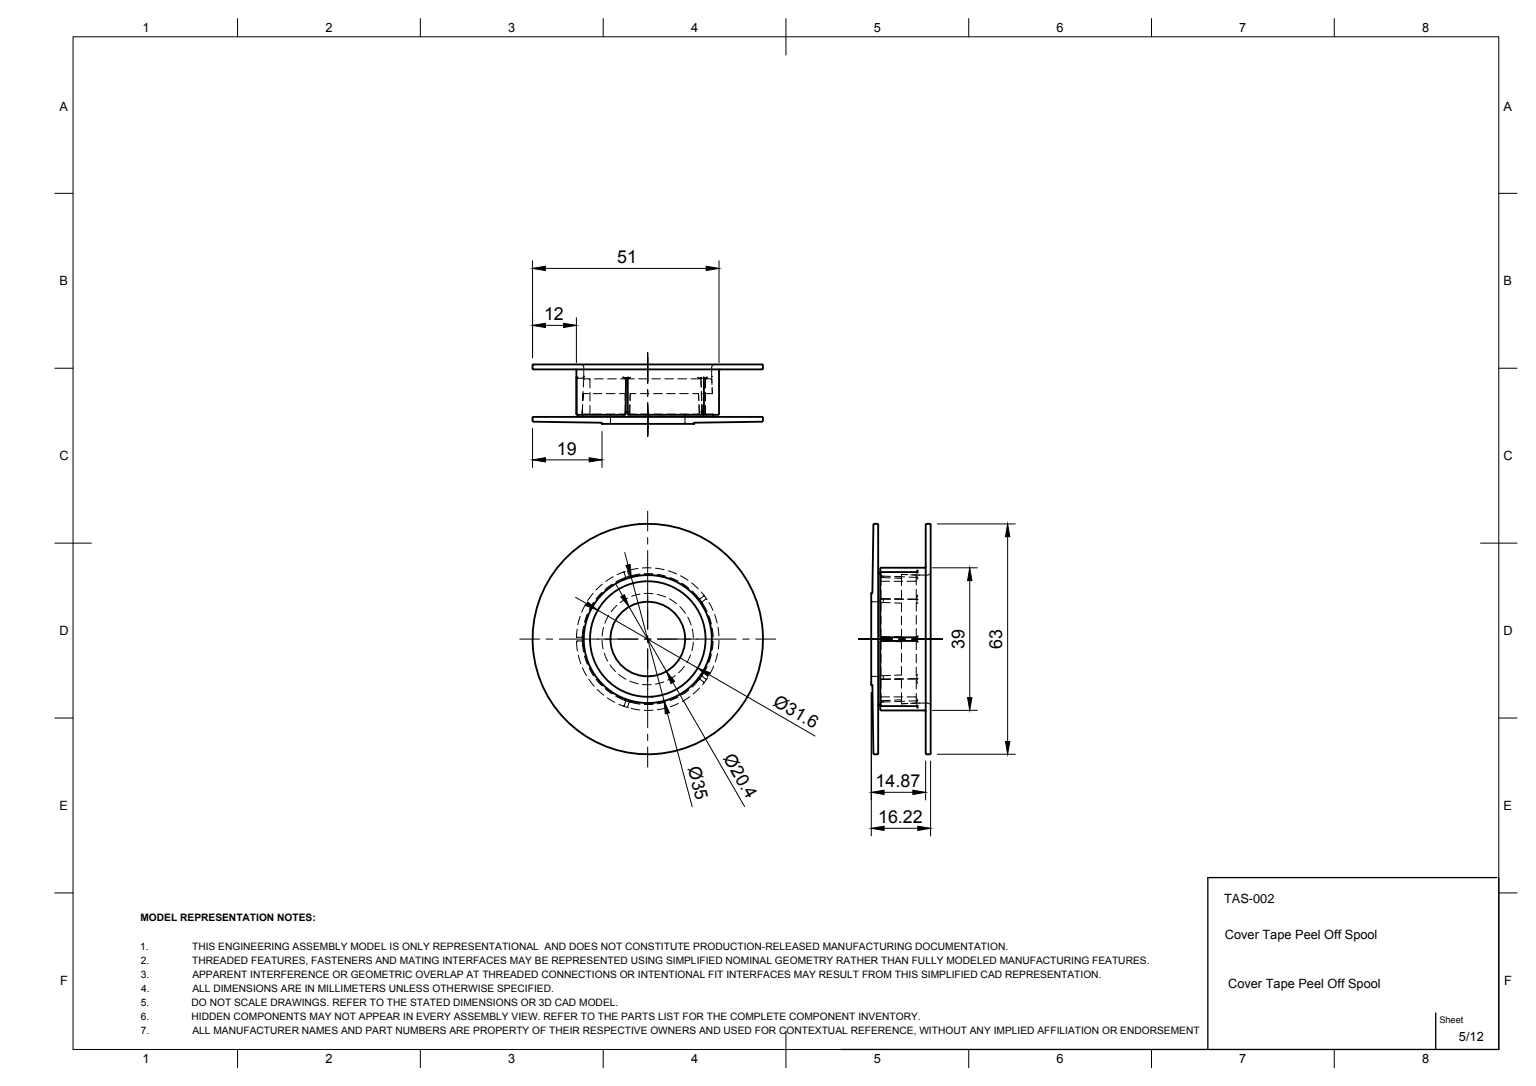
ISO-10303-21;
HEADER;
/* Generated by software containing ST-Developer
 * from STEP Tools, Inc. (www.steptools.com) 
 */

FILE_DESCRIPTION(
/* description */ ('STEP AP214'),
/* implementation_level */ '2;1');

FILE_NAME(
/* name */ 'Cover Tape Peel Off Spool.step',
/* time_stamp */ '2026-11-04T19:38:14-08:00',
/* author */ (''),
/* organization */ (''),
/* preprocessor_version */ 'ST-DEVELOPER v20.2',
/* originating_system */ 'Autodesk Translation Framework v15.17.0.0',
/* authorisation */ '');

FILE_SCHEMA (('AUTOMOTIVE_DESIGN { 1 0 10303 214 3 1 1 }'));
ENDSEC;

DATA;
#10=MECHANICAL_DESIGN_GEOMETRIC_PRESENTATION_REPRESENTATION('',(#472),#36668);
#168=CONICAL_SURFACE('',#18363,17.5,0.0444152152469099);
#169=CONICAL_SURFACE('',#18378,31.5,1.55500816505907);
#170=CONICAL_SURFACE('',#18555,17.5,0.038076825589802);
#193=TOROIDAL_SURFACE('',#18311,15.5,0.3);
#194=TOROIDAL_SURFACE('',#18315,31.2,0.3);
#195=TOROIDAL_SURFACE('',#18320,12.8,0.3);
#196=TOROIDAL_SURFACE('',#18325,10.5,0.3);
#197=TOROIDAL_SURFACE('',#18329,10.5,0.3);
#198=TOROIDAL_SURFACE('',#18334,31.2,0.3);
#199=TOROIDAL_SURFACE('',#18338,18.2,0.3);
#200=TOROIDAL_SURFACE('',#18342,17.2130371832119,0.3);
#201=TOROIDAL_SURFACE('',#18346,16.1,0.3);
#202=TOROIDAL_SURFACE('',#18380,31.25,0.25);
#203=TOROIDAL_SURFACE('',#18385,19.75,0.25);
#204=TOROIDAL_SURFACE('',#18389,17.75,0.25);
#205=TOROIDAL_SURFACE('',#18399,18.1406575306034,0.25);
#206=TOROIDAL_SURFACE('',#18405,19.25,0.25);
#207=TOROIDAL_SURFACE('',#18411,17.759705149651,0.25);
#208=TOROIDAL_SURFACE('',#18414,19.25,0.25);
#209=TOROIDAL_SURFACE('',#18425,17.759705149651,0.25);
#210=TOROIDAL_SURFACE('',#18431,19.25,0.25);
#211=TOROIDAL_SURFACE('',#18435,18.1406575306034,0.25);
#212=TOROIDAL_SURFACE('',#18439,19.25,0.25);
#213=TOROIDAL_SURFACE('',#18452,18.1406575306034,0.25);
#214=TOROIDAL_SURFACE('',#18458,19.25,0.25);
#215=TOROIDAL_SURFACE('',#18462,17.759705149651,0.25);
#216=TOROIDAL_SURFACE('',#18465,19.25,0.25);
#217=TOROIDAL_SURFACE('',#18479,17.759705149651,0.25);
#218=TOROIDAL_SURFACE('',#18485,19.25,0.25);
#219=TOROIDAL_SURFACE('',#18490,18.1406575306034,0.25);
#220=TOROIDAL_SURFACE('',#18493,19.25,0.25);
#221=TOROIDAL_SURFACE('',#18506,18.1406575306034,0.25);
#222=TOROIDAL_SURFACE('',#18513,19.25,0.25);
#223=TOROIDAL_SURFACE('',#18520,17.759705149651,0.25);
#224=TOROIDAL_SURFACE('',#18523,19.25,0.25);
#225=TOROIDAL_SURFACE('',#18530,31.25,0.25);
#226=TOROIDAL_SURFACE('',#18551,18.2999999294072,0.8);
#236=B_SPLINE_CURVE_WITH_KNOTS('',3,(#25581,#25582,#25583,#25584,#25585,
#25586,#25587,#25588,#25589,#25590,#25591,#25592),.UNSPECIFIED.,.F.,.F.,
(4,2,2,2,2,4),(-0.0307505677232343,-0.0290851658458097,-0.0274197639683852,
-0.0256899175968281,-0.0239600712252709,-0.0214016072500974),
 .UNSPECIFIED.);
#237=B_SPLINE_CURVE_WITH_KNOTS('',3,(#25608,#25609,#25610,#25611,#25612,
#25613,#25614,#25615,#25616,#25617,#25618,#25619),.UNSPECIFIED.,.F.,.F.,
(4,2,2,2,2,4),(-0.0400996909613273,-0.0375410642212333,-0.035811217849675,
-0.0340813714781167,-0.0324159696006892,-0.0307505677232617),
 .UNSPECIFIED.);
#238=B_SPLINE_CURVE_WITH_KNOTS('',3,(#25634,#25635,#25636,#25637,#25638,
#25639,#25640,#25641,#25642,#25643,#25644,#25645),.UNSPECIFIED.,.F.,.F.,
(4,2,2,2,2,4),(0.0307505677231893,0.0324159696006138,0.0340813714780383,
0.0358112178495909,0.0375410642211435,0.040099528194227),.UNSPECIFIED.);
#239=B_SPLINE_CURVE_WITH_KNOTS('',3,(#25652,#25653,#25654,#25655,#25656,
#25657,#25658,#25659,#25660,#25661,#25662,#25663),.UNSPECIFIED.,.F.,.F.,
(4,2,2,2,2,4),(0.0214015561623852,0.0239600712252435,0.0256899175967988,
0.0274197639683542,0.0290851658457769,0.0307505677231996),.UNSPECIFIED.);
#240=B_SPLINE_CURVE_WITH_KNOTS('',3,(#25749,#25750,#25751,#25752,#25753,
#25754,#25755,#25756,#25757,#25758,#25759,#25760),.UNSPECIFIED.,.F.,.F.,
(4,2,2,2,2,4),(0.0214014871422872,0.0239600712252674,0.0256899175968258,
0.0274197639683841,0.0290851658458094,0.0307505677232346),.UNSPECIFIED.);
#241=B_SPLINE_CURVE_WITH_KNOTS('',3,(#25762,#25763,#25764,#25765,#25766,
#25767),.UNSPECIFIED.,.F.,.F.,(4,2,4),(0.516167584835576,0.556355629697994,
0.571945746029783),.UNSPECIFIED.);
#242=B_SPLINE_CURVE_WITH_KNOTS('',3,(#25770,#25771,#25772,#25773,#25774,
#25775),.UNSPECIFIED.,.F.,.F.,(4,2,4),(-0.572283818814118,-0.556572033620994,
-0.516504886359884),.UNSPECIFIED.);
#243=B_SPLINE_CURVE_WITH_KNOTS('',3,(#25778,#25779,#25780,#25781,#25782,
#25783),.UNSPECIFIED.,.F.,.F.,(4,2,4),(0.516062927236787,0.556286483365537,
0.571840801367595),.UNSPECIFIED.);
#244=B_SPLINE_CURVE_WITH_KNOTS('',3,(#25787,#25788,#25789,#25790,#25791,
#25792),.UNSPECIFIED.,.F.,.F.,(4,2,4),(-0.572388774164482,-0.556641170070289,
-0.516609564275015),.UNSPECIFIED.);
#245=B_SPLINE_CURVE_WITH_KNOTS('',3,(#25794,#25795,#25796,#25797,#25798,
#25799,#25800,#25801,#25802,#25803,#25804,#25805),.UNSPECIFIED.,.F.,.F.,
(4,2,2,2,2,4),(0.0307505677232594,0.0324159696006859,0.0340813714781124,
0.0358112178496696,0.0375410642212269,0.0400994853939697),.UNSPECIFIED.);
#246=B_SPLINE_CURVE_WITH_KNOTS('',3,(#25809,#25810,#25811,#25812,#25813,
#25814,#25815,#25816,#25817,#25818,#25819,#25820),.UNSPECIFIED.,.F.,.F.,
(4,2,2,2,2,4),(0.0214014871425106,0.0239600712253013,0.0256899175968606,
0.0274197639684198,0.0290851658458467,0.0307505677232736),.UNSPECIFIED.);
#247=B_SPLINE_CURVE_WITH_KNOTS('',3,(#25822,#25823,#25824,#25825,#25826,
#25827),.UNSPECIFIED.,.F.,.F.,(4,2,4),(0.516167584819259,0.556355629663768,
0.571945746013171),.UNSPECIFIED.);
#248=B_SPLINE_CURVE_WITH_KNOTS('',3,(#25830,#25831,#25832,#25833,#25834,
#25835),.UNSPECIFIED.,.F.,.F.,(4,2,4),(-0.572283818796558,-0.556572033600684,
-0.516504886344356),.UNSPECIFIED.);
#249=B_SPLINE_CURVE_WITH_KNOTS('',3,(#25839,#25840,#25841,#25842,#25843,
#25844,#25845,#25846,#25847,#25848,#25849,#25850),.UNSPECIFIED.,.F.,.F.,
(4,2,2,2,2,4),(0.0214015561620376,0.0239600712252775,0.0256899175968367,
0.0274197639683959,0.0290851658458218,0.0307505677232477),.UNSPECIFIED.);
#250=B_SPLINE_CURVE_WITH_KNOTS('',3,(#25852,#25853,#25854,#25855,#25856,
#25857),.UNSPECIFIED.,.F.,.F.,(4,2,4),(0.516336929306378,0.556467476401172,
0.572115549692269),.UNSPECIFIED.);
#251=B_SPLINE_CURVE_WITH_KNOTS('',3,(#25861,#25862,#25863,#25864,#25865,
#25866),.UNSPECIFIED.,.F.,.F.,(4,2,4),(-0.572113997134204,-0.556460133617456,
-0.516335518817303),.UNSPECIFIED.);
#252=B_SPLINE_CURVE_WITH_KNOTS('',3,(#25868,#25869,#25870,#25871,#25872,
#25873,#25874,#25875,#25876,#25877,#25878,#25879),.UNSPECIFIED.,.F.,.F.,
(4,2,2,2,2,4),(0.0307505677232669,0.0324159696006922,0.0340813714781176,
0.0358112178496757,0.0375410642212338,0.0400995974505249),.UNSPECIFIED.);
#253=B_SPLINE_CURVE_WITH_KNOTS('',3,(#25882,#25883,#25884,#25885,#25886,
#25887),.UNSPECIFIED.,.F.,.F.,(4,2,4),(0.516336929316142,0.556467476363535,
0.572115549701707),.UNSPECIFIED.);
#254=B_SPLINE_CURVE_WITH_KNOTS('',3,(#25891,#25892,#25893,#25894,#25895,
#25896),.UNSPECIFIED.,.F.,.F.,(4,2,4),(-0.572087843455165,-0.556460133653863,
-0.516335518814487),.UNSPECIFIED.);
#255=B_SPLINE_CURVE_WITH_KNOTS('',3,(#25898,#25899,#25900,#25901,#25902,
#25903,#25904,#25905,#25906,#25907,#25908,#25909),.UNSPECIFIED.,.F.,.F.,
(4,2,2,2,2,4),(0.0307505677231587,0.0324159696005802,0.0340813714780017,
0.0358112178495531,0.0375410642211044,0.0401277329731923),.UNSPECIFIED.);
#256=B_SPLINE_CURVE_WITH_KNOTS('',3,(#25915,#25916,#25917,#25918,#25919,
#25920,#25921,#25922,#25923,#25924,#25925,#25926,#25927,#25928,#25929,#25930,
#25931,#25932,#25933,#25934,#25935,#25936),.UNSPECIFIED.,.F.,.F.,(4,2,2,
2,2,2,2,2,2,2,4),(2.02457825278125E-10,0.00248408483075073,0.00372612724612612,
0.00434714845381382,0.00465765905765771,0.00481291435957969,0.00489054201054069,
0.00492935583602118,0.00494876274876143,0.00495846620513155,0.00496816966150168),
 .UNSPECIFIED.);
#257=B_SPLINE_CURVE_WITH_KNOTS('',3,(#25938,#25939,#25940,#25941,#25942,
#25943,#25944,#25945,#25946,#25947,#25948,#25949,#25950,#25951,#25952,#25953,
#25954,#25955,#25956,#25957,#25958,#25959),.UNSPECIFIED.,.F.,.F.,(4,2,2,
2,2,2,2,2,2,2,4),(3.5048712953905E-5,4.4761383731225E-5,5.4474054508545E-5,
7.38993960631036E-5,0.00011275007917231,0.000190451445390804,0.000345854177827798,
0.000656659642701783,0.00127827057244967,0.00252149243194545,0.00500793615093709),
 .UNSPECIFIED.);
#258=B_SPLINE_CURVE_WITH_KNOTS('',3,(#25962,#25963,#25964,#25965,#25966,
#25967,#25968,#25969,#25970,#25971,#25972,#25973,#25974,#25975,#25976,#25977,
#25978,#25979,#25980,#25981,#25982,#25983),.UNSPECIFIED.,.F.,.F.,(4,2,2,
2,2,2,2,2,2,2,4),(2.04137276529534E-10,0.00248408522863344,0.00372612784295016,
0.00434714915010856,0.00465765980368776,0.00481291513047741,0.00489054279387223,
0.00492935662556968,0.00494876354141844,0.00495846699934282,0.0049681704572672),
 .UNSPECIFIED.);
#259=B_SPLINE_CURVE_WITH_KNOTS('',3,(#25985,#25986,#25987,#25988,#25989,
#25990,#25991,#25992,#25993,#25994,#25995,#25996,#25997,#25998,#25999,#26000,
#26001,#26002,#26003,#26004,#26005,#26006),.UNSPECIFIED.,.F.,.F.,(4,2,2,
2,2,2,2,2,2,2,4),(3.50520341719619E-5,4.47649965919165E-5,5.44779590118712E-5,
7.3903883851858E-5,0.000112755733531832,0.0001904594328917,0.000345866831611521,
0.000656681629051249,0.00127831122393071,0.00252157041368962,0.00500808879320745),
 .UNSPECIFIED.);
#260=B_SPLINE_CURVE_WITH_KNOTS('',3,(#26014,#26015,#26016,#26017,#26018,
#26019,#26020,#26021,#26022,#26023,#26024,#26025,#26026,#26027,#26028,#26029,
#26030,#26031,#26032,#26033,#26034,#26035),.UNSPECIFIED.,.F.,.F.,(4,2,2,
2,2,2,2,2,2,2,4),(2.06866606511861E-10,0.00248408587267595,0.00372612880901388,
0.00434715027718289,0.00465766101126744,0.00481291637830975,0.00489054406183091,
0.00492935790359148,0.00494876482447177,0.00495846828491192,0.00496817174535206),
 .UNSPECIFIED.);
#261=B_SPLINE_CURVE_WITH_KNOTS('',3,(#26037,#26038,#26039,#26040,#26041,
#26042,#26043,#26044,#26045,#26046,#26047,#26048,#26049,#26050,#26051,#26052,
#26053,#26054,#26055,#26056,#26057,#26058),.UNSPECIFIED.,.F.,.F.,(4,2,2,
2,2,2,2,2,2,2,4),(3.50574081053878E-5,4.47708507809905E-5,5.44842934565933E-5,
7.39111788077861E-5,0.000112764949510167,0.000190472490915007,0.000345887573724691,
0.000656717739344059,0.00127837807058271,0.00252169873306001,0.00500834005801461),
 .UNSPECIFIED.);
#262=B_SPLINE_CURVE_WITH_KNOTS('',3,(#26061,#26062,#26063,#26064,#26065,
#26066,#26067,#26068,#26069,#26070,#26071,#26072,#26073,#26074,#26075,#26076,
#26077,#26078,#26079,#26080,#26081,#26082),.UNSPECIFIED.,.F.,.F.,(4,2,2,
2,2,2,2,2,2,2,4),(2.06867445612259E-10,0.00248408587267104,0.00372612880900657,
0.00434715027717433,0.00465766101125817,0.00481291637830013,0.00489054406182111,
0.0049293579035816,0.00494876482446188,0.00495846828490199,0.00496817174534209),
 .UNSPECIFIED.);
#263=B_SPLINE_CURVE_WITH_KNOTS('',3,(#26084,#26085,#26086,#26087,#26088,
#26089,#26090,#26091,#26092,#26093,#26094,#26095,#26096,#26097,#26098,#26099,
#26100,#26101,#26102,#26103,#26104,#26105),.UNSPECIFIED.,.F.,.F.,(4,2,2,
2,2,2,2,2,2,2,4),(3.50574081266199E-5,4.47708505998206E-5,5.44842930730214E-5,
7.39111780194308E-5,0.000112764947912246,0.000190472487697963,0.000345887567269397,
0.000656717726412263,0.001278378044698,0.00252169868126955,0.00500833995441257),
 .UNSPECIFIED.);
#264=B_SPLINE_CURVE_WITH_KNOTS('',3,(#26108,#26109,#26110,#26111,#26112,
#26113,#26114,#26115,#26116,#26117,#26118,#26119,#26120,#26121,#26122,#26123,
#26124,#26125,#26126,#26127,#26128,#26129),.UNSPECIFIED.,.F.,.F.,(4,2,2,
2,2,2,2,2,2,2,4),(2.04137059199594E-10,0.00248408522863389,0.00372612784295087,
0.00434714915010935,0.00465765980368859,0.00481291513047817,0.00489054279387297,
0.00492935662557032,0.00494876354141895,0.00495846699934332,0.00496817045726768),
 .UNSPECIFIED.);
#265=B_SPLINE_CURVE_WITH_KNOTS('',3,(#26130,#26131,#26132,#26133,#26134,
#26135,#26136,#26137,#26138,#26139,#26140,#26141,#26142,#26143,#26144,#26145,
#26146,#26147,#26148,#26149,#26150,#26151),.UNSPECIFIED.,.F.,.F.,(4,2,2,
2,2,2,2,2,2,2,4),(3.50520341720812E-5,4.47649965026772E-5,5.44779588332732E-5,
7.39038834943838E-5,0.000112755732816681,0.00019045943146128,0.000345866828750562,
0.00065668162332904,0.00127831121248599,0.00252157039079989,0.00500808874742778),
 .UNSPECIFIED.);
#266=B_SPLINE_CURVE_WITH_KNOTS('',3,(#26205,#26206,#26207,#26208,#26209,
#26210,#26211,#26212,#26213,#26214,#26215,#26216,#26217,#26218),
 .UNSPECIFIED.,.F.,.F.,(4,2,2,2,2,2,4),(-0.000304965314045538,0.,0.000936499595052828,
0.00576011793928687,0.00947606916598535,0.0122802204486003,0.0139854910646116),
 .UNSPECIFIED.);
#267=B_SPLINE_CURVE_WITH_KNOTS('',3,(#26225,#26226,#26227,#26228,#26229,
#26230,#26231,#26232,#26233,#26234,#26235,#26236,#26237,#26238,#26239,#26240),
 .UNSPECIFIED.,.F.,.F.,(4,2,2,2,2,2,2,4),(0.0536858997421767,0.0538805473387552,
0.0625727109542441,0.0725640535967514,0.0859159770081403,0.0987536985065928,
0.112218387900172,0.112607088674662),.UNSPECIFIED.);
#268=B_SPLINE_CURVE_WITH_KNOTS('',3,(#26255,#26256,#26257,#26258,#26259,
#26260,#26261,#26262,#26263,#26264,#26265,#26266,#26267,#26268,#26269,#26270),
 .UNSPECIFIED.,.F.,.F.,(4,2,2,2,2,2,2,4),(-0.0122740412193648,-0.0121759293582432,
-0.0120897396500415,-0.0111319415843575,-0.00947389246986148,-0.00820108783558479,
-0.0071868786468098,-0.00688693855294442),.UNSPECIFIED.);
#269=B_SPLINE_CURVE_WITH_KNOTS('',3,(#26276,#26277,#26278,#26279,#26280,
#26281,#26282,#26283,#26284,#26285,#26286,#26287,#26288,#26289,#26290,#26291),
 .UNSPECIFIED.,.F.,.F.,(4,2,2,2,2,2,2,4),(-0.0477691295327812,-0.0476102750821729,
-0.0405164866112679,-0.0323624211355981,-0.0214657417184032,-0.0109887092110674,
0.,0.000317223788085325),.UNSPECIFIED.);
#270=B_SPLINE_CURVE_WITH_KNOTS('',3,(#26303,#26304,#26305,#26306,#26307,
#26308,#26309,#26310,#26311,#26312,#26313,#26314,#26315,#26316,#26317,#26318),
 .UNSPECIFIED.,.F.,.F.,(4,2,2,2,2,2,2,4),(0.00685142344086609,0.00716754606670829,
0.00817883021840179,0.00945159950065682,0.0111102560598908,0.0126000677878647,
0.0134555802450022,0.0143116650403246),.UNSPECIFIED.);
#271=B_SPLINE_CURVE_WITH_KNOTS('',3,(#26340,#26341,#26342,#26343,#26344,
#26345,#26346,#26347,#26348,#26349,#26350,#26351,#26352,#26353,#26354,#26355),
 .UNSPECIFIED.,.F.,.F.,(4,2,2,2,2,2,2,4),(-0.000317223787690337,3.02215934569472E-15,
0.0109887092111399,0.0214657417185508,0.0323624211357588,0.0405164866114483,
0.0476102750823548,0.047769129532989),.UNSPECIFIED.);
#272=B_SPLINE_CURVE_WITH_KNOTS('',3,(#26359,#26360,#26361,#26362,#26363,
#26364,#26365,#26366,#26367,#26368,#26369,#26370,#26371,#26372),
 .UNSPECIFIED.,.F.,.F.,(4,2,2,2,2,2,4),(-0.0138875980614929,-0.0121989286884961,
-0.00941634599982081,-0.00572975137256096,-0.00094390537822651,0.,0.000305060128611046),
 .UNSPECIFIED.);
#273=B_SPLINE_CURVE_WITH_KNOTS('',3,(#26384,#26385,#26386,#26387,#26388,
#26389,#26390,#26391,#26392,#26393,#26394,#26395,#26396,#26397,#26398,#26399),
 .UNSPECIFIED.,.F.,.F.,(4,2,2,2,2,2,2,4),(-0.112607088625168,-0.112218387851368,
-0.0987536984648267,-0.0859159769729998,-0.0725640535676872,-0.0625727109298437,
-0.0538805473185267,-0.053685899721448),.UNSPECIFIED.);
#274=B_SPLINE_CURVE_WITH_KNOTS('',3,(#26440,#26441,#26442,#26443,#26444,
#26445,#26446,#26447,#26448,#26449,#26450,#26451,#26452,#26453),
 .UNSPECIFIED.,.F.,.F.,(4,2,2,2,2,2,4),(-0.000304965268692175,0.,0.000936496117482782,
0.00576013224595397,0.00947609729856078,0.0122802587445126,0.0139855371807907),
 .UNSPECIFIED.);
#275=B_SPLINE_CURVE_WITH_KNOTS('',3,(#26463,#26464,#26465,#26466,#26467,
#26468,#26469,#26470,#26471,#26472,#26473,#26474,#26475,#26476,#26477,#26478),
 .UNSPECIFIED.,.F.,.F.,(4,2,2,2,2,2,2,4),(0.0536858997392164,0.0538805473358447,
0.0625727109506776,0.072564053592395,0.0859159770028611,0.0987536985002761,
0.112218387892815,0.112607088666955),.UNSPECIFIED.);
#276=B_SPLINE_CURVE_WITH_KNOTS('',3,(#26492,#26493,#26494,#26495,#26496,
#26497,#26498,#26499,#26500,#26501,#26502,#26503,#26504,#26505,#26506,#26507),
 .UNSPECIFIED.,.F.,.F.,(4,2,2,2,2,2,2,4),(-0.0122740769336355,-0.0121759644410632,
-0.0120897737524462,-0.0111319575392944,-0.00947390765146132,-0.00820110219546828,
-0.00718689112173828,-0.00688695772759274),.UNSPECIFIED.);
#277=B_SPLINE_CURVE_WITH_KNOTS('',3,(#26513,#26514,#26515,#26516,#26517,
#26518,#26519,#26520,#26521,#26522,#26523,#26524,#26525,#26526,#26527,#26528),
 .UNSPECIFIED.,.F.,.F.,(4,2,2,2,2,2,2,4),(-0.0477691295328705,-0.0476102750818484,
-0.0405164866108641,-0.0323624211350328,-0.0214657417175428,-0.0109887092105592,
0.,0.00031722378862325),.UNSPECIFIED.);
#278=B_SPLINE_CURVE_WITH_KNOTS('',3,(#26544,#26545,#26546,#26547,#26548,
#26549,#26550,#26551,#26552,#26553,#26554,#26555,#26556,#26557,#26558,#26559),
 .UNSPECIFIED.,.F.,.F.,(4,2,2,2,2,2,2,4),(0.00683098498387795,0.00715685727468737,
0.0081665770863791,0.0094395668715797,0.0110988523787266,0.0125271081563038,
0.0131709865966103,0.0138210554549785),.UNSPECIFIED.);
#279=B_SPLINE_CURVE_WITH_KNOTS('',3,(#26580,#26581,#26582,#26583,#26584,
#26585,#26586,#26587,#26588,#26589,#26590,#26591,#26592,#26593,#26594,#26595),
 .UNSPECIFIED.,.F.,.F.,(4,2,2,2,2,2,2,4),(-0.000317223788318669,0.,0.0109887092111283,
0.0214657417185403,0.0323624211358337,0.0405164866115566,0.0476102750824874,
0.0477691295331555),.UNSPECIFIED.);
#280=B_SPLINE_CURVE_WITH_KNOTS('',3,(#26599,#26600,#26601,#26602,#26603,
#26604,#26605,#26606,#26607,#26608,#26609,#26610,#26611,#26612),
 .UNSPECIFIED.,.F.,.F.,(4,2,2,2,2,2,4),(-0.013826978099047,-0.0121485991715528,
-0.00937937937785604,-0.00571097373361621,-0.000948519651099016,0.,0.00030511843446065),
 .UNSPECIFIED.);
#281=B_SPLINE_CURVE_WITH_KNOTS('',3,(#26624,#26625,#26626,#26627,#26628,
#26629,#26630,#26631,#26632,#26633,#26634,#26635,#26636,#26637,#26638,#26639),
 .UNSPECIFIED.,.F.,.F.,(4,2,2,2,2,2,2,4),(-0.112607088663875,-0.112218387889847,
-0.0987536984976824,-0.0859159770006442,-0.0725640535905707,-0.0625727109491047,
-0.0538805473344791,-0.0536858997378307),.UNSPECIFIED.);
#282=B_SPLINE_CURVE_WITH_KNOTS('',3,(#26682,#26683,#26684,#26685,#26686,
#26687,#26688,#26689,#26690,#26691,#26692,#26693,#26694,#26695),
 .UNSPECIFIED.,.F.,.F.,(4,2,2,2,2,2,4),(-0.00030506004969664,0.,0.000943899264666623,
0.00572977625979271,0.0094163950019481,0.012198995415075,0.0138876784363644),
 .UNSPECIFIED.);
#283=B_SPLINE_CURVE_WITH_KNOTS('',3,(#26705,#26706,#26707,#26708,#26709,
#26710,#26711,#26712,#26713,#26714,#26715,#26716,#26717,#26718,#26719,#26720),
 .UNSPECIFIED.,.F.,.F.,(4,2,2,2,2,2,2,4),(0.0536858997405358,0.053880547337153,
0.0625727109524208,0.072564053594619,0.0859159770056253,0.0987536985036731,
0.112218387896803,0.112607088671311),.UNSPECIFIED.);
#284=B_SPLINE_CURVE_WITH_KNOTS('',3,(#26737,#26738,#26739,#26740,#26741,
#26742,#26743,#26744,#26745,#26746,#26747,#26748,#26749,#26750,#26751,#26752),
 .UNSPECIFIED.,.F.,.F.,(4,2,2,2,2,2,2,4),(-0.0143120844458313,-0.0134558136848229,
-0.0126001113738633,-0.0111102618619966,-0.00945160573383406,-0.00817883662994094,
-0.00716755165087691,-0.00685143448301955),.UNSPECIFIED.);
#285=B_SPLINE_CURVE_WITH_KNOTS('',3,(#26758,#26759,#26760,#26761,#26762,
#26763,#26764,#26765,#26766,#26767,#26768,#26769,#26770,#26771,#26772,#26773),
 .UNSPECIFIED.,.F.,.F.,(4,2,2,2,2,2,2,4),(-0.0477691295329166,-0.0476102750829768,
-0.0405164866121143,-0.0323624211366189,-0.0214657417197341,-0.0109887092118291,
0.,0.000317223787610884),.UNSPECIFIED.);
#387=SPHERICAL_SURFACE('',#18271,0.25);
#388=SPHERICAL_SURFACE('',#18275,0.25);
#389=SPHERICAL_SURFACE('',#18279,0.25);
#390=SPHERICAL_SURFACE('',#18283,0.25);
#391=SPHERICAL_SURFACE('',#18287,0.25);
#392=SPHERICAL_SURFACE('',#18291,0.25);
#393=SPHERICAL_SURFACE('',#18295,0.25);
#394=SPHERICAL_SURFACE('',#18299,0.25);
#395=SPHERICAL_SURFACE('',#18303,0.25);
#396=SPHERICAL_SURFACE('',#18307,0.25);
#397=SPHERICAL_SURFACE('',#18396,0.25);
#398=SPHERICAL_SURFACE('',#18408,0.25);
#399=SPHERICAL_SURFACE('',#18428,0.25);
#400=SPHERICAL_SURFACE('',#18445,0.25);
#401=SPHERICAL_SURFACE('',#18448,0.25);
#402=SPHERICAL_SURFACE('',#18468,0.25);
#403=SPHERICAL_SURFACE('',#18482,0.25);
#404=SPHERICAL_SURFACE('',#18499,0.25);
#405=SPHERICAL_SURFACE('',#18502,0.25);
#406=SPHERICAL_SURFACE('',#18517,0.25);
#452=SHAPE_REPRESENTATION_RELATIONSHIP('SRR','None',#36708,#462);
#462=ADVANCED_BREP_SHAPE_REPRESENTATION('',(#482),#36660);
#472=STYLED_ITEM('',(#36767),#482);
#482=MANIFOLD_SOLID_BREP('Body1',#17795);
#547=CYLINDRICAL_SURFACE('',#18350,31.5);
#548=CYLINDRICAL_SURFACE('',#18351,17.9);
#549=CYLINDRICAL_SURFACE('',#18372,15.8);
#550=CYLINDRICAL_SURFACE('',#18374,10.2);
#551=CYLINDRICAL_SURFACE('',#18377,12.5);
#552=CYLINDRICAL_SURFACE('',#18394,0.250000000000003);
#553=CYLINDRICAL_SURFACE('',#18402,0.249999569584526);
#554=CYLINDRICAL_SURFACE('',#18403,0.249999999999998);
#555=CYLINDRICAL_SURFACE('',#18417,0.250000000000003);
#556=CYLINDRICAL_SURFACE('',#18418,0.249999570396522);
#557=CYLINDRICAL_SURFACE('',#18419,0.249999576130625);
#558=CYLINDRICAL_SURFACE('',#18420,0.249999999999998);
#559=CYLINDRICAL_SURFACE('',#18423,0.249999999999998);
#560=CYLINDRICAL_SURFACE('',#18434,0.249999575380867);
#561=CYLINDRICAL_SURFACE('',#18438,0.250000000000003);
#562=CYLINDRICAL_SURFACE('',#18442,0.249999999999998);
#563=CYLINDRICAL_SURFACE('',#18451,0.250000000000003);
#564=CYLINDRICAL_SURFACE('',#18454,0.249999569575431);
#565=CYLINDRICAL_SURFACE('',#18455,0.249999999999998);
#566=CYLINDRICAL_SURFACE('',#18456,0.249999999999998);
#567=CYLINDRICAL_SURFACE('',#18471,0.250000000000006);
#568=CYLINDRICAL_SURFACE('',#18472,0.249999566833149);
#569=CYLINDRICAL_SURFACE('',#18473,0.24999957614651);
#570=CYLINDRICAL_SURFACE('',#18475,0.249999999999998);
#571=CYLINDRICAL_SURFACE('',#18477,0.249999999999996);
#572=CYLINDRICAL_SURFACE('',#18488,0.249999578947113);
#573=CYLINDRICAL_SURFACE('',#18492,0.249999999999998);
#574=CYLINDRICAL_SURFACE('',#18497,0.249999999999996);
#575=CYLINDRICAL_SURFACE('',#18505,0.250000000000006);
#576=CYLINDRICAL_SURFACE('',#18509,0.249999575366884);
#577=CYLINDRICAL_SURFACE('',#18510,0.250000000000004);
#578=CYLINDRICAL_SURFACE('',#18511,0.250000000000004);
#579=CYLINDRICAL_SURFACE('',#18526,0.250000000000004);
#580=CYLINDRICAL_SURFACE('',#18527,0.249999570396437);
#581=CYLINDRICAL_SURFACE('',#18528,0.250000000000004);
#582=CYLINDRICAL_SURFACE('',#18554,17.5);
#583=CYLINDRICAL_SURFACE('',#18557,19.5);
#584=CYLINDRICAL_SURFACE('',#18559,31.5);
#885=FACE_BOUND('',#2822,.T.);
#886=FACE_BOUND('',#2825,.T.);
#887=FACE_BOUND('',#2828,.T.);
#888=FACE_BOUND('',#2832,.T.);
#889=FACE_BOUND('',#2913,.T.);
#890=FACE_BOUND('',#2920,.T.);
#1083=CIRCLE('',#18272,0.250000000000003);
#1084=CIRCLE('',#18273,0.249999999999998);
#1085=CIRCLE('',#18274,0.250000000000004);
#1086=CIRCLE('',#18276,0.249999999999996);
#1087=CIRCLE('',#18277,0.25);
#1088=CIRCLE('',#18278,0.249999999999993);
#1089=CIRCLE('',#18280,0.249999999999998);
#1090=CIRCLE('',#18281,0.250000000000003);
#1091=CIRCLE('',#18282,0.250000000000001);
#1092=CIRCLE('',#18284,0.249999999999998);
#1093=CIRCLE('',#18285,0.249999999999997);
#1094=CIRCLE('',#18286,0.249999999999998);
#1095=CIRCLE('',#18288,0.250000000000002);
#1096=CIRCLE('',#18289,0.250000000000006);
#1097=CIRCLE('',#18290,0.25);
#1098=CIRCLE('',#18292,0.249999999999995);
#1099=CIRCLE('',#18293,0.249999999999998);
#1100=CIRCLE('',#18294,0.249999999999998);
#1101=CIRCLE('',#18296,0.250000000000003);
#1102=CIRCLE('',#18297,0.249999999999997);
#1103=CIRCLE('',#18298,0.250000000000005);
#1104=CIRCLE('',#18300,0.250000000000004);
#1105=CIRCLE('',#18301,0.25);
#1106=CIRCLE('',#18302,0.249999999999998);
#1107=CIRCLE('',#18304,0.249999999999998);
#1108=CIRCLE('',#18305,0.250000000000003);
#1109=CIRCLE('',#18306,0.250000000000007);
#1110=CIRCLE('',#18308,0.250000000000005);
#1111=CIRCLE('',#18309,0.250000000000003);
#1112=CIRCLE('',#18310,0.249999999999998);
#1113=CIRCLE('',#18312,15.8);
#1114=CIRCLE('',#18313,0.3);
#1115=CIRCLE('',#18314,15.5);
#1116=CIRCLE('',#18316,31.5);
#1117=CIRCLE('',#18317,31.5);
#1118=CIRCLE('',#18318,0.3);
#1119=CIRCLE('',#18319,31.2047362517505);
#1120=CIRCLE('',#18321,12.5);
#1121=CIRCLE('',#18322,0.3);
#1122=CIRCLE('',#18323,12.7952637482494);
#1123=CIRCLE('',#18324,12.7952637482494);
#1124=CIRCLE('',#18326,10.5);
#1125=CIRCLE('',#18327,0.3);
#1126=CIRCLE('',#18328,10.2);
#1127=CIRCLE('',#18330,10.5);
#1128=CIRCLE('',#18331,0.3);
#1129=CIRCLE('',#18332,10.2);
#1130=CIRCLE('',#18333,10.2);
#1131=CIRCLE('',#18335,31.5);
#1132=CIRCLE('',#18336,0.3);
#1133=CIRCLE('',#18337,31.2);
#1134=CIRCLE('',#18339,18.2);
#1135=CIRCLE('',#18340,0.3);
#1136=CIRCLE('',#18341,17.9);
#1137=CIRCLE('',#18343,17.5127413251518);
#1138=CIRCLE('',#18344,0.3);
#1139=CIRCLE('',#18345,17.2130371832119);
#1140=CIRCLE('',#18347,16.1);
#1141=CIRCLE('',#18348,0.3);
#1142=CIRCLE('',#18349,15.8);
#1143=CIRCLE('',#18352,17.9);
#1144=CIRCLE('',#18353,17.9);
#1145=CIRCLE('',#18354,17.9);
#1146=CIRCLE('',#18355,17.9);
#1147=CIRCLE('',#18356,17.9);
#1148=CIRCLE('',#18357,17.9);
#1149=CIRCLE('',#18358,17.9);
#1150=CIRCLE('',#18359,17.9);
#1151=CIRCLE('',#18360,17.9);
#1152=CIRCLE('',#18361,17.9);
#1153=CIRCLE('',#18362,17.9);
#1154=CIRCLE('',#18364,17.6796049747715);
#1155=CIRCLE('',#18365,17.6796049747715);
#1156=CIRCLE('',#18366,17.6796049747715);
#1157=CIRCLE('',#18367,17.6796049747715);
#1158=CIRCLE('',#18368,17.6796049747715);
#1159=CIRCLE('',#18369,17.6796049747715);
#1160=CIRCLE('',#18370,17.6796049747715);
#1161=CIRCLE('',#18376,12.5);
#1162=CIRCLE('',#18381,31.5);
#1163=CIRCLE('',#18382,31.5);
#1164=CIRCLE('',#18383,0.25);
#1165=CIRCLE('',#18384,31.25);
#1166=CIRCLE('',#18386,19.75);
#1167=CIRCLE('',#18387,0.25);
#1168=CIRCLE('',#18388,19.5);
#1169=CIRCLE('',#18390,17.5);
#1170=CIRCLE('',#18391,17.5);
#1171=CIRCLE('',#18392,0.25);
#1172=CIRCLE('',#18393,17.5001812086856);
#1173=CIRCLE('',#18395,0.250000000000003);
#1174=CIRCLE('',#18397,0.250000000000004);
#1175=CIRCLE('',#18398,0.249999999999994);
#1176=CIRCLE('',#18400,18.1406575306034);
#1177=CIRCLE('',#18401,0.250000000000002);
#1178=CIRCLE('',#18404,0.249999999999998);
#1179=CIRCLE('',#18406,19.25);
#1180=CIRCLE('',#18407,19.5);
#1181=CIRCLE('',#18409,0.250000000000001);
#1182=CIRCLE('',#18410,0.250000000000003);
#1183=CIRCLE('',#18412,17.759705149651);
#1184=CIRCLE('',#18413,17.5098863583366);
#1185=CIRCLE('',#18415,19.5);
#1186=CIRCLE('',#18416,19.25);
#1187=CIRCLE('',#18421,0.249999999999998);
#1188=CIRCLE('',#18422,0.249999999999998);
#1189=CIRCLE('',#18424,0.249999999999998);
#1190=CIRCLE('',#18426,17.5098863583366);
#1191=CIRCLE('',#18427,17.759705149651);
#1192=CIRCLE('',#18429,0.249999999999995);
#1193=CIRCLE('',#18430,0.250000000000003);
#1194=CIRCLE('',#18432,19.25);
#1195=CIRCLE('',#18433,19.5);
#1196=CIRCLE('',#18436,0.249999999999993);
#1197=CIRCLE('',#18437,18.1406575306034);
#1198=CIRCLE('',#18440,19.5);
#1199=CIRCLE('',#18441,19.25);
#1200=CIRCLE('',#18443,0.249999999999998);
#1201=CIRCLE('',#18444,0.249999999999998);
#1202=CIRCLE('',#18446,0.249999999999999);
#1203=CIRCLE('',#18447,0.25);
#1204=CIRCLE('',#18449,0.250000000000003);
#1205=CIRCLE('',#18450,0.250000000000005);
#1206=CIRCLE('',#18453,18.1406575306034);
#1207=CIRCLE('',#18457,0.249999999999998);
#1208=CIRCLE('',#18459,0.250000000000002);
#1209=CIRCLE('',#18460,19.25);
#1210=CIRCLE('',#18461,19.5);
#1211=CIRCLE('',#18463,17.759705149651);
#1212=CIRCLE('',#18464,17.5098863583366);
#1213=CIRCLE('',#18466,19.5);
#1214=CIRCLE('',#18467,19.25);
#1215=CIRCLE('',#18469,0.249999999999996);
#1216=CIRCLE('',#18470,0.250000000000006);
#1217=CIRCLE('',#18474,0.249999999999999);
#1218=CIRCLE('',#18476,0.249999999999998);
#1219=CIRCLE('',#18478,0.249999999999996);
#1220=CIRCLE('',#18480,17.5098863583366);
#1221=CIRCLE('',#18481,17.759705149651);
#1222=CIRCLE('',#18483,0.249999999999997);
#1223=CIRCLE('',#18484,0.249999999999998);
#1224=CIRCLE('',#18486,19.25);
#1225=CIRCLE('',#18487,19.5);
#1226=CIRCLE('',#18489,0.250000000000002);
#1227=CIRCLE('',#18491,18.1406575306034);
#1228=CIRCLE('',#18494,0.250000000000001);
#1229=CIRCLE('',#18495,19.5);
#1230=CIRCLE('',#18496,19.25);
#1231=CIRCLE('',#18498,0.249999999999996);
#1232=CIRCLE('',#18500,0.250000000000004);
#1233=CIRCLE('',#18501,0.250000000000006);
#1234=CIRCLE('',#18503,0.250000000000004);
#1235=CIRCLE('',#18504,0.250000000000004);
#1236=CIRCLE('',#18507,18.1406575306034);
#1237=CIRCLE('',#18508,0.250000000000003);
#1238=CIRCLE('',#18512,0.250000000000004);
#1239=CIRCLE('',#18514,19.25);
#1240=CIRCLE('',#18515,19.5);
#1241=CIRCLE('',#18516,19.5);
#1242=CIRCLE('',#18518,0.250000000000004);
#1243=CIRCLE('',#18519,0.25);
#1244=CIRCLE('',#18521,17.759705149651);
#1245=CIRCLE('',#18522,17.5098863583366);
#1246=CIRCLE('',#18524,19.5);
#1247=CIRCLE('',#18525,19.25);
#1248=CIRCLE('',#18529,0.250000000000004);
#1249=CIRCLE('',#18531,31.5);
#1250=CIRCLE('',#18532,0.25);
#1251=CIRCLE('',#18533,31.25);
#1252=CIRCLE('',#18550,18.2999999762315);
#1253=CIRCLE('',#18552,17.5);
#1254=CIRCLE('',#18553,0.8);
#1759=FACE_OUTER_BOUND('',#2799,.T.);
#1760=FACE_OUTER_BOUND('',#2800,.T.);
#1761=FACE_OUTER_BOUND('',#2801,.T.);
#1762=FACE_OUTER_BOUND('',#2802,.T.);
#1763=FACE_OUTER_BOUND('',#2803,.T.);
#1764=FACE_OUTER_BOUND('',#2804,.T.);
#1765=FACE_OUTER_BOUND('',#2805,.T.);
#1766=FACE_OUTER_BOUND('',#2806,.T.);
#1767=FACE_OUTER_BOUND('',#2807,.T.);
#1768=FACE_OUTER_BOUND('',#2808,.T.);
#1769=FACE_OUTER_BOUND('',#2809,.T.);
#1770=FACE_OUTER_BOUND('',#2810,.T.);
#1771=FACE_OUTER_BOUND('',#2811,.T.);
#1772=FACE_OUTER_BOUND('',#2812,.T.);
#1773=FACE_OUTER_BOUND('',#2813,.T.);
#1774=FACE_OUTER_BOUND('',#2814,.T.);
#1775=FACE_OUTER_BOUND('',#2815,.T.);
#1776=FACE_OUTER_BOUND('',#2816,.T.);
#1777=FACE_OUTER_BOUND('',#2817,.T.);
#1778=FACE_OUTER_BOUND('',#2818,.T.);
#1779=FACE_OUTER_BOUND('',#2819,.T.);
#1780=FACE_OUTER_BOUND('',#2820,.T.);
#1781=FACE_OUTER_BOUND('',#2821,.T.);
#1782=FACE_OUTER_BOUND('',#2823,.T.);
#1783=FACE_OUTER_BOUND('',#2824,.T.);
#1784=FACE_OUTER_BOUND('',#2826,.T.);
#1785=FACE_OUTER_BOUND('',#2827,.T.);
#1786=FACE_OUTER_BOUND('',#2829,.T.);
#1787=FACE_OUTER_BOUND('',#2830,.T.);
#1788=FACE_OUTER_BOUND('',#2831,.T.);
#1789=FACE_OUTER_BOUND('',#2833,.T.);
#1790=FACE_OUTER_BOUND('',#2834,.T.);
#1791=FACE_OUTER_BOUND('',#2835,.T.);
#1792=FACE_OUTER_BOUND('',#2836,.T.);
#1793=FACE_OUTER_BOUND('',#2837,.T.);
#1794=FACE_OUTER_BOUND('',#2838,.T.);
#1795=FACE_OUTER_BOUND('',#2839,.T.);
#1796=FACE_OUTER_BOUND('',#2840,.T.);
#1797=FACE_OUTER_BOUND('',#2841,.T.);
#1798=FACE_OUTER_BOUND('',#2842,.T.);
#1799=FACE_OUTER_BOUND('',#2843,.T.);
#1800=FACE_OUTER_BOUND('',#2844,.T.);
#1801=FACE_OUTER_BOUND('',#2845,.T.);
#1802=FACE_OUTER_BOUND('',#2846,.T.);
#1803=FACE_OUTER_BOUND('',#2847,.T.);
#1804=FACE_OUTER_BOUND('',#2848,.T.);
#1805=FACE_OUTER_BOUND('',#2849,.T.);
#1806=FACE_OUTER_BOUND('',#2850,.T.);
#1807=FACE_OUTER_BOUND('',#2851,.T.);
#1808=FACE_OUTER_BOUND('',#2852,.T.);
#1809=FACE_OUTER_BOUND('',#2853,.T.);
#1810=FACE_OUTER_BOUND('',#2854,.T.);
#1811=FACE_OUTER_BOUND('',#2855,.T.);
#1812=FACE_OUTER_BOUND('',#2856,.T.);
#1813=FACE_OUTER_BOUND('',#2857,.T.);
#1814=FACE_OUTER_BOUND('',#2858,.T.);
#1815=FACE_OUTER_BOUND('',#2859,.T.);
#1816=FACE_OUTER_BOUND('',#2860,.T.);
#1817=FACE_OUTER_BOUND('',#2861,.T.);
#1818=FACE_OUTER_BOUND('',#2862,.T.);
#1819=FACE_OUTER_BOUND('',#2863,.T.);
#1820=FACE_OUTER_BOUND('',#2864,.T.);
#1821=FACE_OUTER_BOUND('',#2865,.T.);
#1822=FACE_OUTER_BOUND('',#2866,.T.);
#1823=FACE_OUTER_BOUND('',#2867,.T.);
#1824=FACE_OUTER_BOUND('',#2868,.T.);
#1825=FACE_OUTER_BOUND('',#2869,.T.);
#1826=FACE_OUTER_BOUND('',#2870,.T.);
#1827=FACE_OUTER_BOUND('',#2871,.T.);
#1828=FACE_OUTER_BOUND('',#2872,.T.);
#1829=FACE_OUTER_BOUND('',#2873,.T.);
#1830=FACE_OUTER_BOUND('',#2874,.T.);
#1831=FACE_OUTER_BOUND('',#2875,.T.);
#1832=FACE_OUTER_BOUND('',#2876,.T.);
#1833=FACE_OUTER_BOUND('',#2877,.T.);
#1834=FACE_OUTER_BOUND('',#2878,.T.);
#1835=FACE_OUTER_BOUND('',#2879,.T.);
#1836=FACE_OUTER_BOUND('',#2880,.T.);
#1837=FACE_OUTER_BOUND('',#2881,.T.);
#1838=FACE_OUTER_BOUND('',#2882,.T.);
#1839=FACE_OUTER_BOUND('',#2883,.T.);
#1840=FACE_OUTER_BOUND('',#2884,.T.);
#1841=FACE_OUTER_BOUND('',#2885,.T.);
#1842=FACE_OUTER_BOUND('',#2886,.T.);
#1843=FACE_OUTER_BOUND('',#2887,.T.);
#1844=FACE_OUTER_BOUND('',#2888,.T.);
#1845=FACE_OUTER_BOUND('',#2889,.T.);
#1846=FACE_OUTER_BOUND('',#2890,.T.);
#1847=FACE_OUTER_BOUND('',#2891,.T.);
#1848=FACE_OUTER_BOUND('',#2892,.T.);
#1849=FACE_OUTER_BOUND('',#2893,.T.);
#1850=FACE_OUTER_BOUND('',#2894,.T.);
#1851=FACE_OUTER_BOUND('',#2895,.T.);
#1852=FACE_OUTER_BOUND('',#2896,.T.);
#1853=FACE_OUTER_BOUND('',#2897,.T.);
#1854=FACE_OUTER_BOUND('',#2898,.T.);
#1855=FACE_OUTER_BOUND('',#2899,.T.);
#1856=FACE_OUTER_BOUND('',#2900,.T.);
#1857=FACE_OUTER_BOUND('',#2901,.T.);
#1858=FACE_OUTER_BOUND('',#2902,.T.);
#1859=FACE_OUTER_BOUND('',#2903,.T.);
#1860=FACE_OUTER_BOUND('',#2904,.T.);
#1861=FACE_OUTER_BOUND('',#2905,.T.);
#1862=FACE_OUTER_BOUND('',#2906,.T.);
#1863=FACE_OUTER_BOUND('',#2907,.T.);
#1864=FACE_OUTER_BOUND('',#2908,.T.);
#1865=FACE_OUTER_BOUND('',#2909,.T.);
#1866=FACE_OUTER_BOUND('',#2910,.T.);
#1867=FACE_OUTER_BOUND('',#2911,.T.);
#1868=FACE_OUTER_BOUND('',#2912,.T.);
#1869=FACE_OUTER_BOUND('',#2914,.T.);
#1870=FACE_OUTER_BOUND('',#2915,.T.);
#1871=FACE_OUTER_BOUND('',#2916,.T.);
#1872=FACE_OUTER_BOUND('',#2917,.T.);
#1873=FACE_OUTER_BOUND('',#2918,.T.);
#1874=FACE_OUTER_BOUND('',#2919,.T.);
#1875=FACE_OUTER_BOUND('',#2921,.T.);
#1876=FACE_OUTER_BOUND('',#2922,.T.);
#1877=FACE_OUTER_BOUND('',#2923,.T.);
#1878=FACE_OUTER_BOUND('',#2924,.T.);
#1879=FACE_OUTER_BOUND('',#2925,.T.);
#2799=EDGE_LOOP('',(#12562,#12563,#12564));
#2800=EDGE_LOOP('',(#12565,#12566,#12567));
#2801=EDGE_LOOP('',(#12568,#12569,#12570,#12571));
#2802=EDGE_LOOP('',(#12572,#12573,#12574));
#2803=EDGE_LOOP('',(#12575,#12576,#12577,#12578));
#2804=EDGE_LOOP('',(#12579,#12580,#12581));
#2805=EDGE_LOOP('',(#12582,#12583,#12584,#12585));
#2806=EDGE_LOOP('',(#12586,#12587,#12588,#12589));
#2807=EDGE_LOOP('',(#12590,#12591,#12592));
#2808=EDGE_LOOP('',(#12593,#12594,#12595));
#2809=EDGE_LOOP('',(#12596,#12597,#12598,#12599));
#2810=EDGE_LOOP('',(#12600,#12601,#12602,#12603,#12604));
#2811=EDGE_LOOP('',(#12605,#12606,#12607,#12608,#12609));
#2812=EDGE_LOOP('',(#12610,#12611,#12612,#12613));
#2813=EDGE_LOOP('',(#12614,#12615,#12616,#12617,#12618));
#2814=EDGE_LOOP('',(#12619,#12620,#12621,#12622));
#2815=EDGE_LOOP('',(#12623,#12624,#12625,#12626));
#2816=EDGE_LOOP('',(#12627,#12628,#12629,#12630));
#2817=EDGE_LOOP('',(#12631,#12632,#12633,#12634));
#2818=EDGE_LOOP('',(#12635,#12636,#12637,#12638,#12639));
#2819=EDGE_LOOP('',(#12640,#12641,#12642,#12643,#12644,#12645,#12646,#12647,
#12648,#12649,#12650,#12651,#12652,#12653,#12654,#12655,#12656,#12657,#12658,
#12659,#12660,#12661,#12662,#12663,#12664,#12665,#12666,#12667,#12668,#12669,
#12670,#12671,#12672,#12673));
#2820=EDGE_LOOP('',(#12674,#12675,#12676,#12677,#12678,#12679,#12680,#12681,
#12682,#12683,#12684,#12685,#12686,#12687,#12688,#12689,#12690,#12691,#12692,
#12693,#12694,#12695,#12696,#12697,#12698));
#2821=EDGE_LOOP('',(#12699));
#2822=EDGE_LOOP('',(#12700));
#2823=EDGE_LOOP('',(#12701,#12702,#12703,#12704));
#2824=EDGE_LOOP('',(#12705));
#2825=EDGE_LOOP('',(#12706));
#2826=EDGE_LOOP('',(#12707,#12708,#12709,#12710,#12711));
#2827=EDGE_LOOP('',(#12712));
#2828=EDGE_LOOP('',(#12713));
#2829=EDGE_LOOP('',(#12714,#12715,#12716,#12717));
#2830=EDGE_LOOP('',(#12718,#12719,#12720,#12721,#12722));
#2831=EDGE_LOOP('',(#12723));
#2832=EDGE_LOOP('',(#12724));
#2833=EDGE_LOOP('',(#12725,#12726,#12727,#12728,#12729));
#2834=EDGE_LOOP('',(#12730,#12731,#12732,#12733));
#2835=EDGE_LOOP('',(#12734,#12735,#12736,#12737,#12738));
#2836=EDGE_LOOP('',(#12739,#12740,#12741,#12742));
#2837=EDGE_LOOP('',(#12743,#12744,#12745,#12746));
#2838=EDGE_LOOP('',(#12747,#12748,#12749,#12750,#12751));
#2839=EDGE_LOOP('',(#12752,#12753,#12754,#12755,#12756,#12757,#12758));
#2840=EDGE_LOOP('',(#12759,#12760,#12761,#12762,#12763));
#2841=EDGE_LOOP('',(#12764,#12765,#12766,#12767));
#2842=EDGE_LOOP('',(#12768,#12769,#12770,#12771));
#2843=EDGE_LOOP('',(#12772,#12773,#12774,#12775));
#2844=EDGE_LOOP('',(#12776,#12777,#12778,#12779));
#2845=EDGE_LOOP('',(#12780,#12781,#12782,#12783));
#2846=EDGE_LOOP('',(#12784,#12785,#12786,#12787,#12788,#12789,#12790));
#2847=EDGE_LOOP('',(#12791,#12792,#12793,#12794,#12795,#12796,#12797));
#2848=EDGE_LOOP('',(#12798,#12799,#12800,#12801,#12802));
#2849=EDGE_LOOP('',(#12803,#12804,#12805,#12806,#12807));
#2850=EDGE_LOOP('',(#12808,#12809,#12810,#12811));
#2851=EDGE_LOOP('',(#12812,#12813,#12814));
#2852=EDGE_LOOP('',(#12815,#12816,#12817,#12818));
#2853=EDGE_LOOP('',(#12819,#12820,#12821,#12822,#12823,#12824,#12825));
#2854=EDGE_LOOP('',(#12826,#12827,#12828,#12829));
#2855=EDGE_LOOP('',(#12830,#12831,#12832,#12833));
#2856=EDGE_LOOP('',(#12834,#12835,#12836,#12837));
#2857=EDGE_LOOP('',(#12838,#12839,#12840,#12841,#12842));
#2858=EDGE_LOOP('',(#12843,#12844,#12845,#12846));
#2859=EDGE_LOOP('',(#12847,#12848,#12849));
#2860=EDGE_LOOP('',(#12850,#12851,#12852,#12853));
#2861=EDGE_LOOP('',(#12854,#12855,#12856,#12857));
#2862=EDGE_LOOP('',(#12858,#12859,#12860,#12861,#12862,#12863,#12864));
#2863=EDGE_LOOP('',(#12865,#12866,#12867,#12868));
#2864=EDGE_LOOP('',(#12869,#12870,#12871,#12872,#12873));
#2865=EDGE_LOOP('',(#12874,#12875,#12876,#12877));
#2866=EDGE_LOOP('',(#12878,#12879,#12880,#12881));
#2867=EDGE_LOOP('',(#12882,#12883,#12884,#12885));
#2868=EDGE_LOOP('',(#12886,#12887,#12888));
#2869=EDGE_LOOP('',(#12889,#12890,#12891,#12892));
#2870=EDGE_LOOP('',(#12893,#12894,#12895,#12896,#12897,#12898,#12899));
#2871=EDGE_LOOP('',(#12900,#12901,#12902,#12903,#12904,#12905,#12906));
#2872=EDGE_LOOP('',(#12907,#12908,#12909,#12910,#12911));
#2873=EDGE_LOOP('',(#12912,#12913,#12914,#12915,#12916));
#2874=EDGE_LOOP('',(#12917,#12918,#12919,#12920));
#2875=EDGE_LOOP('',(#12921,#12922,#12923,#12924));
#2876=EDGE_LOOP('',(#12925,#12926,#12927,#12928));
#2877=EDGE_LOOP('',(#12929,#12930,#12931,#12932,#12933,#12934,#12935));
#2878=EDGE_LOOP('',(#12936,#12937,#12938,#12939));
#2879=EDGE_LOOP('',(#12940,#12941,#12942,#12943));
#2880=EDGE_LOOP('',(#12944,#12945,#12946,#12947));
#2881=EDGE_LOOP('',(#12948,#12949,#12950,#12951,#12952));
#2882=EDGE_LOOP('',(#12953,#12954,#12955,#12956));
#2883=EDGE_LOOP('',(#12957,#12958,#12959));
#2884=EDGE_LOOP('',(#12960,#12961,#12962,#12963));
#2885=EDGE_LOOP('',(#12964,#12965,#12966,#12967));
#2886=EDGE_LOOP('',(#12968,#12969,#12970,#12971,#12972,#12973,#12974));
#2887=EDGE_LOOP('',(#12975,#12976,#12977,#12978));
#2888=EDGE_LOOP('',(#12979,#12980,#12981,#12982,#12983));
#2889=EDGE_LOOP('',(#12984,#12985,#12986,#12987,#12988));
#2890=EDGE_LOOP('',(#12989,#12990,#12991,#12992));
#2891=EDGE_LOOP('',(#12993,#12994,#12995,#12996));
#2892=EDGE_LOOP('',(#12997,#12998,#12999,#13000));
#2893=EDGE_LOOP('',(#13001,#13002,#13003,#13004));
#2894=EDGE_LOOP('',(#13005,#13006,#13007,#13008,#13009,#13010,#13011));
#2895=EDGE_LOOP('',(#13012,#13013,#13014,#13015,#13016));
#2896=EDGE_LOOP('',(#13017,#13018,#13019,#13020));
#2897=EDGE_LOOP('',(#13021,#13022,#13023,#13024,#13025,#13026,#13027,#13028));
#2898=EDGE_LOOP('',(#13029,#13030,#13031,#13032));
#2899=EDGE_LOOP('',(#13033,#13034,#13035,#13036));
#2900=EDGE_LOOP('',(#13037,#13038,#13039,#13040,#13041,#13042,#13043,#13044));
#2901=EDGE_LOOP('',(#13045,#13046,#13047,#13048));
#2902=EDGE_LOOP('',(#13049,#13050,#13051,#13052));
#2903=EDGE_LOOP('',(#13053,#13054,#13055,#13056,#13057,#13058,#13059,#13060));
#2904=EDGE_LOOP('',(#13061,#13062,#13063,#13064));
#2905=EDGE_LOOP('',(#13065,#13066,#13067,#13068));
#2906=EDGE_LOOP('',(#13069,#13070,#13071,#13072,#13073,#13074,#13075,#13076));
#2907=EDGE_LOOP('',(#13077,#13078,#13079,#13080));
#2908=EDGE_LOOP('',(#13081,#13082,#13083,#13084));
#2909=EDGE_LOOP('',(#13085,#13086,#13087,#13088,#13089,#13090,#13091,#13092));
#2910=EDGE_LOOP('',(#13093,#13094,#13095,#13096));
#2911=EDGE_LOOP('',(#13097,#13098,#13099,#13100));
#2912=EDGE_LOOP('',(#13101));
#2913=EDGE_LOOP('',(#13102));
#2914=EDGE_LOOP('',(#13103,#13104,#13105,#13106));
#2915=EDGE_LOOP('',(#13107,#13108,#13109,#13110,#13111));
#2916=EDGE_LOOP('',(#13112,#13113,#13114,#13115,#13116,#13117,#13118,#13119,
#13120,#13121,#13122,#13123,#13124,#13125,#13126,#13127,#13128,#13129,#13130,
#13131,#13132,#13133,#13134,#13135,#13136));
#2917=EDGE_LOOP('',(#13137,#13138,#13139,#13140));
#2918=EDGE_LOOP('',(#13141,#13142,#13143,#13144,#13145,#13146,#13147,#13148,
#13149,#13150,#13151,#13152,#13153,#13154,#13155,#13156,#13157,#13158,#13159,
#13160,#13161,#13162,#13163,#13164));
#2919=EDGE_LOOP('',(#13165));
#2920=EDGE_LOOP('',(#13166));
#2921=EDGE_LOOP('',(#13167,#13168,#13169,#13170,#13171));
#2922=EDGE_LOOP('',(#13172,#13173,#13174,#13175));
#2923=EDGE_LOOP('',(#13176,#13177,#13178,#13179));
#2924=EDGE_LOOP('',(#13180,#13181,#13182,#13183));
#2925=EDGE_LOOP('',(#13184,#13185,#13186,#13187));
#4138=LINE('',#25742,#5848);
#4139=LINE('',#25745,#5849);
#4140=LINE('',#26011,#5850);
#4141=LINE('',#26154,#5851);
#4142=LINE('',#26157,#5852);
#4143=LINE('',#26162,#5853);
#4144=LINE('',#26164,#5854);
#4145=LINE('',#26190,#5855);
#4146=LINE('',#26193,#5856);
#4147=LINE('',#26203,#5857);
#4148=LINE('',#26220,#5858);
#4149=LINE('',#26221,#5859);
#4150=LINE('',#26241,#5860);
#4151=LINE('',#26243,#5861);
#4152=LINE('',#26295,#5862);
#4153=LINE('',#26296,#5863);
#4154=LINE('',#26299,#5864);
#4155=LINE('',#26301,#5865);
#4156=LINE('',#26319,#5866);
#4157=LINE('',#26321,#5867);
#4158=LINE('',#26323,#5868);
#4159=LINE('',#26324,#5869);
#4160=LINE('',#26329,#5870);
#4161=LINE('',#26332,#5871);
#4162=LINE('',#26337,#5872);
#4163=LINE('',#26339,#5873);
#4164=LINE('',#26401,#5874);
#4165=LINE('',#26403,#5875);
#4166=LINE('',#26404,#5876);
#4167=LINE('',#26410,#5877);
#4168=LINE('',#26411,#5878);
#4169=LINE('',#26420,#5879);
#4170=LINE('',#26422,#5880);
#4171=LINE('',#26432,#5881);
#4172=LINE('',#26433,#5882);
#4173=LINE('',#26438,#5883);
#4174=LINE('',#26455,#5884);
#4175=LINE('',#26456,#5885);
#4176=LINE('',#26458,#5886);
#4177=LINE('',#26459,#5887);
#4178=LINE('',#26479,#5888);
#4179=LINE('',#26481,#5889);
#4180=LINE('',#26536,#5890);
#4181=LINE('',#26537,#5891);
#4182=LINE('',#26540,#5892);
#4183=LINE('',#26542,#5893);
#4184=LINE('',#26560,#5894);
#4185=LINE('',#26562,#5895);
#4186=LINE('',#26566,#5896);
#4187=LINE('',#26567,#5897);
#4188=LINE('',#26569,#5898);
#4189=LINE('',#26572,#5899);
#4190=LINE('',#26577,#5900);
#4191=LINE('',#26579,#5901);
#4192=LINE('',#26643,#5902);
#4193=LINE('',#26645,#5903);
#4194=LINE('',#26646,#5904);
#4195=LINE('',#26650,#5905);
#4196=LINE('',#26651,#5906);
#4197=LINE('',#26660,#5907);
#4198=LINE('',#26662,#5908);
#4199=LINE('',#26672,#5909);
#4200=LINE('',#26673,#5910);
#4201=LINE('',#26680,#5911);
#4202=LINE('',#26697,#5912);
#4203=LINE('',#26698,#5913);
#4204=LINE('',#26700,#5914);
#4205=LINE('',#26701,#5915);
#4206=LINE('',#26721,#5916);
#4207=LINE('',#26723,#5917);
#4208=LINE('',#26777,#5918);
#4209=LINE('',#26778,#5919);
#4210=LINE('',#26780,#5920);
#4211=LINE('',#26782,#5921);
#4212=LINE('',#26783,#5922);
#4213=LINE('',#26787,#5923);
#4214=LINE('',#26788,#5924);
#4215=LINE('',#26796,#5925);
#4216=LINE('',#26797,#5926);
#4217=LINE('',#26801,#5927);
#4218=LINE('',#26802,#5928);
#4219=LINE('',#26806,#5929);
#4220=LINE('',#26807,#5930);
#4221=LINE('',#26811,#5931);
#4222=LINE('',#26812,#5932);
#4223=LINE('',#26816,#5933);
#4224=LINE('',#26817,#5934);
#4225=LINE('',#26828,#5935);
#4226=LINE('',#26830,#5936);
#4227=LINE('',#26833,#5937);
#4228=LINE('',#26836,#5938);
#5848=VECTOR('',#20862,31.5);
#5849=VECTOR('',#20865,17.9);
#5850=VECTOR('',#20898,17.5);
#5851=VECTOR('',#20909,15.8);
#5852=VECTOR('',#20914,10.2);
#5853=VECTOR('',#20921,12.5);
#5854=VECTOR('',#20924,31.5);
#5855=VECTOR('',#20957,1000.);
#5856=VECTOR('',#20960,1000.);
#5857=VECTOR('',#20975,10.);
#5858=VECTOR('',#20976,10.);
#5859=VECTOR('',#20977,10.);
#5860=VECTOR('',#20980,1000.);
#5861=VECTOR('',#20981,1000.);
#5862=VECTOR('',#21010,1000.);
#5863=VECTOR('',#21011,1000.);
#5864=VECTOR('',#21014,10.);
#5865=VECTOR('',#21015,10.);
#5866=VECTOR('',#21016,10.);
#5867=VECTOR('',#21019,10.);
#5868=VECTOR('',#21020,10.);
#5869=VECTOR('',#21021,10.);
#5870=VECTOR('',#21026,1000.);
#5871=VECTOR('',#21029,1000.);
#5872=VECTOR('',#21034,1000.);
#5873=VECTOR('',#21035,1000.);
#5874=VECTOR('',#21056,10.);
#5875=VECTOR('',#21057,10.);
#5876=VECTOR('',#21058,10.);
#5877=VECTOR('',#21067,1000.);
#5878=VECTOR('',#21068,1000.);
#5879=VECTOR('',#21079,1000.);
#5880=VECTOR('',#21082,1000.);
#5881=VECTOR('',#21097,1000.);
#5882=VECTOR('',#21098,1000.);
#5883=VECTOR('',#21105,10.);
#5884=VECTOR('',#21106,10.);
#5885=VECTOR('',#21107,10.);
#5886=VECTOR('',#21110,1000.);
#5887=VECTOR('',#21111,1000.);
#5888=VECTOR('',#21114,1000.);
#5889=VECTOR('',#21115,1000.);
#5890=VECTOR('',#21146,1000.);
#5891=VECTOR('',#21147,1000.);
#5892=VECTOR('',#21150,10.);
#5893=VECTOR('',#21151,10.);
#5894=VECTOR('',#21152,10.);
#5895=VECTOR('',#21155,10.);
#5896=VECTOR('',#21158,10.);
#5897=VECTOR('',#21159,10.);
#5898=VECTOR('',#21162,1000.);
#5899=VECTOR('',#21165,1000.);
#5900=VECTOR('',#21170,1000.);
#5901=VECTOR('',#21171,1000.);
#5902=VECTOR('',#21194,10.);
#5903=VECTOR('',#21195,10.);
#5904=VECTOR('',#21196,10.);
#5905=VECTOR('',#21203,1000.);
#5906=VECTOR('',#21204,1000.);
#5907=VECTOR('',#21215,1000.);
#5908=VECTOR('',#21218,1000.);
#5909=VECTOR('',#21233,1000.);
#5910=VECTOR('',#21234,1000.);
#5911=VECTOR('',#21243,10.);
#5912=VECTOR('',#21244,10.);
#5913=VECTOR('',#21245,10.);
#5914=VECTOR('',#21248,1000.);
#5915=VECTOR('',#21249,1000.);
#5916=VECTOR('',#21252,1000.);
#5917=VECTOR('',#21253,1000.);
#5918=VECTOR('',#21284,1000.);
#5919=VECTOR('',#21285,1000.);
#5920=VECTOR('',#21288,10.);
#5921=VECTOR('',#21289,10.);
#5922=VECTOR('',#21290,10.);
#5923=VECTOR('',#21295,1000.);
#5924=VECTOR('',#21296,1000.);
#5925=VECTOR('',#21307,1000.);
#5926=VECTOR('',#21308,1000.);
#5927=VECTOR('',#21315,1000.);
#5928=VECTOR('',#21316,1000.);
#5929=VECTOR('',#21323,1000.);
#5930=VECTOR('',#21324,1000.);
#5931=VECTOR('',#21331,1000.);
#5932=VECTOR('',#21332,1000.);
#5933=VECTOR('',#21339,1000.);
#5934=VECTOR('',#21340,1000.);
#5935=VECTOR('',#21357,17.5);
#5936=VECTOR('',#21360,17.5);
#5937=VECTOR('',#21365,19.5);
#5938=VECTOR('',#21370,31.5);
#7445=VERTEX_POINT('',#25560);
#7446=VERTEX_POINT('',#25561);
#7447=VERTEX_POINT('',#25563);
#7448=VERTEX_POINT('',#25567);
#7449=VERTEX_POINT('',#25568);
#7450=VERTEX_POINT('',#25570);
#7451=VERTEX_POINT('',#25574);
#7452=VERTEX_POINT('',#25575);
#7453=VERTEX_POINT('',#25577);
#7454=VERTEX_POINT('',#25579);
#7455=VERTEX_POINT('',#25594);
#7456=VERTEX_POINT('',#25595);
#7457=VERTEX_POINT('',#25597);
#7458=VERTEX_POINT('',#25601);
#7459=VERTEX_POINT('',#25602);
#7460=VERTEX_POINT('',#25604);
#7461=VERTEX_POINT('',#25606);
#7462=VERTEX_POINT('',#25621);
#7463=VERTEX_POINT('',#25622);
#7464=VERTEX_POINT('',#25624);
#7465=VERTEX_POINT('',#25628);
#7466=VERTEX_POINT('',#25629);
#7467=VERTEX_POINT('',#25631);
#7468=VERTEX_POINT('',#25633);
#7469=VERTEX_POINT('',#25648);
#7470=VERTEX_POINT('',#25649);
#7471=VERTEX_POINT('',#25651);
#7472=VERTEX_POINT('',#25664);
#7473=VERTEX_POINT('',#25668);
#7474=VERTEX_POINT('',#25669);
#7475=VERTEX_POINT('',#25671);
#7476=VERTEX_POINT('',#25675);
#7477=VERTEX_POINT('',#25676);
#7478=VERTEX_POINT('',#25678);
#7479=VERTEX_POINT('',#25682);
#7480=VERTEX_POINT('',#25684);
#7481=VERTEX_POINT('',#25688);
#7482=VERTEX_POINT('',#25689);
#7483=VERTEX_POINT('',#25692);
#7484=VERTEX_POINT('',#25696);
#7485=VERTEX_POINT('',#25698);
#7486=VERTEX_POINT('',#25700);
#7487=VERTEX_POINT('',#25704);
#7488=VERTEX_POINT('',#25706);
#7489=VERTEX_POINT('',#25710);
#7490=VERTEX_POINT('',#25712);
#7491=VERTEX_POINT('',#25714);
#7492=VERTEX_POINT('',#25718);
#7493=VERTEX_POINT('',#25720);
#7494=VERTEX_POINT('',#25724);
#7495=VERTEX_POINT('',#25726);
#7496=VERTEX_POINT('',#25730);
#7497=VERTEX_POINT('',#25732);
#7498=VERTEX_POINT('',#25736);
#7499=VERTEX_POINT('',#25738);
#7500=VERTEX_POINT('',#25744);
#7501=VERTEX_POINT('',#25746);
#7502=VERTEX_POINT('',#25748);
#7503=VERTEX_POINT('',#25761);
#7504=VERTEX_POINT('',#25768);
#7505=VERTEX_POINT('',#25777);
#7506=VERTEX_POINT('',#25784);
#7507=VERTEX_POINT('',#25786);
#7508=VERTEX_POINT('',#25793);
#7509=VERTEX_POINT('',#25806);
#7510=VERTEX_POINT('',#25808);
#7511=VERTEX_POINT('',#25821);
#7512=VERTEX_POINT('',#25828);
#7513=VERTEX_POINT('',#25836);
#7514=VERTEX_POINT('',#25838);
#7515=VERTEX_POINT('',#25851);
#7516=VERTEX_POINT('',#25858);
#7517=VERTEX_POINT('',#25860);
#7518=VERTEX_POINT('',#25867);
#7519=VERTEX_POINT('',#25881);
#7520=VERTEX_POINT('',#25888);
#7521=VERTEX_POINT('',#25890);
#7522=VERTEX_POINT('',#25897);
#7523=VERTEX_POINT('',#25912);
#7524=VERTEX_POINT('',#25913);
#7525=VERTEX_POINT('',#25937);
#7526=VERTEX_POINT('',#25960);
#7527=VERTEX_POINT('',#25984);
#7528=VERTEX_POINT('',#26007);
#7529=VERTEX_POINT('',#26009);
#7530=VERTEX_POINT('',#26012);
#7531=VERTEX_POINT('',#26036);
#7532=VERTEX_POINT('',#26059);
#7533=VERTEX_POINT('',#26083);
#7534=VERTEX_POINT('',#26106);
#7535=VERTEX_POINT('',#26159);
#7536=VERTEX_POINT('',#26167);
#7537=VERTEX_POINT('',#26168);
#7538=VERTEX_POINT('',#26171);
#7539=VERTEX_POINT('',#26175);
#7540=VERTEX_POINT('',#26177);
#7541=VERTEX_POINT('',#26181);
#7542=VERTEX_POINT('',#26182);
#7543=VERTEX_POINT('',#26185);
#7544=VERTEX_POINT('',#26189);
#7545=VERTEX_POINT('',#26191);
#7546=VERTEX_POINT('',#26198);
#7547=VERTEX_POINT('',#26202);
#7548=VERTEX_POINT('',#26204);
#7549=VERTEX_POINT('',#26219);
#7550=VERTEX_POINT('',#26223);
#7551=VERTEX_POINT('',#26224);
#7552=VERTEX_POINT('',#26242);
#7553=VERTEX_POINT('',#26249);
#7554=VERTEX_POINT('',#26253);
#7555=VERTEX_POINT('',#26254);
#7556=VERTEX_POINT('',#26274);
#7557=VERTEX_POINT('',#26275);
#7558=VERTEX_POINT('',#26298);
#7559=VERTEX_POINT('',#26300);
#7560=VERTEX_POINT('',#26302);
#7561=VERTEX_POINT('',#26322);
#7562=VERTEX_POINT('',#26326);
#7563=VERTEX_POINT('',#26327);
#7564=VERTEX_POINT('',#26330);
#7565=VERTEX_POINT('',#26334);
#7566=VERTEX_POINT('',#26335);
#7567=VERTEX_POINT('',#26338);
#7568=VERTEX_POINT('',#26357);
#7569=VERTEX_POINT('',#26358);
#7570=VERTEX_POINT('',#26376);
#7571=VERTEX_POINT('',#26380);
#7572=VERTEX_POINT('',#26382);
#7573=VERTEX_POINT('',#26402);
#7574=VERTEX_POINT('',#26406);
#7575=VERTEX_POINT('',#26416);
#7576=VERTEX_POINT('',#26417);
#7577=VERTEX_POINT('',#26419);
#7578=VERTEX_POINT('',#26424);
#7579=VERTEX_POINT('',#26428);
#7580=VERTEX_POINT('',#26437);
#7581=VERTEX_POINT('',#26439);
#7582=VERTEX_POINT('',#26454);
#7583=VERTEX_POINT('',#26461);
#7584=VERTEX_POINT('',#26462);
#7585=VERTEX_POINT('',#26480);
#7586=VERTEX_POINT('',#26484);
#7587=VERTEX_POINT('',#26485);
#7588=VERTEX_POINT('',#26490);
#7589=VERTEX_POINT('',#26491);
#7590=VERTEX_POINT('',#26511);
#7591=VERTEX_POINT('',#26512);
#7592=VERTEX_POINT('',#26532);
#7593=VERTEX_POINT('',#26539);
#7594=VERTEX_POINT('',#26541);
#7595=VERTEX_POINT('',#26543);
#7596=VERTEX_POINT('',#26563);
#7597=VERTEX_POINT('',#26565);
#7598=VERTEX_POINT('',#26570);
#7599=VERTEX_POINT('',#26574);
#7600=VERTEX_POINT('',#26575);
#7601=VERTEX_POINT('',#26578);
#7602=VERTEX_POINT('',#26597);
#7603=VERTEX_POINT('',#26598);
#7604=VERTEX_POINT('',#26616);
#7605=VERTEX_POINT('',#26620);
#7606=VERTEX_POINT('',#26622);
#7607=VERTEX_POINT('',#26641);
#7608=VERTEX_POINT('',#26644);
#7609=VERTEX_POINT('',#26653);
#7610=VERTEX_POINT('',#26654);
#7611=VERTEX_POINT('',#26659);
#7612=VERTEX_POINT('',#26664);
#7613=VERTEX_POINT('',#26668);
#7614=VERTEX_POINT('',#26675);
#7615=VERTEX_POINT('',#26679);
#7616=VERTEX_POINT('',#26681);
#7617=VERTEX_POINT('',#26696);
#7618=VERTEX_POINT('',#26703);
#7619=VERTEX_POINT('',#26704);
#7620=VERTEX_POINT('',#26722);
#7621=VERTEX_POINT('',#26727);
#7622=VERTEX_POINT('',#26731);
#7623=VERTEX_POINT('',#26735);
#7624=VERTEX_POINT('',#26736);
#7625=VERTEX_POINT('',#26756);
#7626=VERTEX_POINT('',#26757);
#7627=VERTEX_POINT('',#26781);
#7628=VERTEX_POINT('',#26785);
#7629=VERTEX_POINT('',#26790);
#7630=VERTEX_POINT('',#26792);
#7631=VERTEX_POINT('',#26821);
#7632=VERTEX_POINT('',#26824);
#9333=EDGE_CURVE('',#7445,#7446,#1083,.T.);
#9334=EDGE_CURVE('',#7447,#7446,#1084,.T.);
#9335=EDGE_CURVE('',#7447,#7445,#1085,.T.);
#9336=EDGE_CURVE('',#7448,#7449,#1086,.T.);
#9337=EDGE_CURVE('',#7448,#7450,#1087,.T.);
#9338=EDGE_CURVE('',#7450,#7449,#1088,.T.);
#9339=EDGE_CURVE('',#7451,#7452,#1089,.T.);
#9340=EDGE_CURVE('',#7452,#7453,#1090,.T.);
#9341=EDGE_CURVE('',#7454,#7453,#1091,.T.);
#9342=EDGE_CURVE('',#7454,#7451,#236,.T.);
#9343=EDGE_CURVE('',#7455,#7456,#1092,.T.);
#9344=EDGE_CURVE('',#7456,#7457,#1093,.T.);
#9345=EDGE_CURVE('',#7455,#7457,#1094,.T.);
#9346=EDGE_CURVE('',#7458,#7459,#1095,.T.);
#9347=EDGE_CURVE('',#7458,#7460,#1096,.T.);
#9348=EDGE_CURVE('',#7460,#7461,#1097,.T.);
#9349=EDGE_CURVE('',#7461,#7459,#237,.T.);
#9350=EDGE_CURVE('',#7462,#7463,#1098,.T.);
#9351=EDGE_CURVE('',#7462,#7464,#1099,.T.);
#9352=EDGE_CURVE('',#7464,#7463,#1100,.T.);
#9353=EDGE_CURVE('',#7465,#7466,#1101,.T.);
#9354=EDGE_CURVE('',#7466,#7467,#1102,.T.);
#9355=EDGE_CURVE('',#7467,#7468,#238,.T.);
#9356=EDGE_CURVE('',#7465,#7468,#1103,.T.);
#9357=EDGE_CURVE('',#7469,#7470,#1104,.T.);
#9358=EDGE_CURVE('',#7469,#7471,#239,.T.);
#9359=EDGE_CURVE('',#7471,#7472,#1105,.T.);
#9360=EDGE_CURVE('',#7472,#7470,#1106,.T.);
#9361=EDGE_CURVE('',#7473,#7474,#1107,.T.);
#9362=EDGE_CURVE('',#7474,#7475,#1108,.T.);
#9363=EDGE_CURVE('',#7473,#7475,#1109,.T.);
#9364=EDGE_CURVE('',#7476,#7477,#1110,.T.);
#9365=EDGE_CURVE('',#7478,#7477,#1111,.T.);
#9366=EDGE_CURVE('',#7478,#7476,#1112,.T.);
#9367=EDGE_CURVE('',#7479,#7479,#1113,.T.);
#9368=EDGE_CURVE('',#7479,#7480,#1114,.T.);
#9369=EDGE_CURVE('',#7480,#7480,#1115,.T.);
#9370=EDGE_CURVE('',#7481,#7482,#1116,.T.);
#9371=EDGE_CURVE('',#7482,#7481,#1117,.T.);
#9372=EDGE_CURVE('',#7482,#7483,#1118,.T.);
#9373=EDGE_CURVE('',#7483,#7483,#1119,.T.);
#9374=EDGE_CURVE('',#7484,#7484,#1120,.T.);
#9375=EDGE_CURVE('',#7484,#7485,#1121,.T.);
#9376=EDGE_CURVE('',#7486,#7485,#1122,.T.);
#9377=EDGE_CURVE('',#7485,#7486,#1123,.T.);
#9378=EDGE_CURVE('',#7487,#7487,#1124,.T.);
#9379=EDGE_CURVE('',#7487,#7488,#1125,.T.);
#9380=EDGE_CURVE('',#7488,#7488,#1126,.T.);
#9381=EDGE_CURVE('',#7489,#7489,#1127,.T.);
#9382=EDGE_CURVE('',#7489,#7490,#1128,.T.);
#9383=EDGE_CURVE('',#7491,#7490,#1129,.T.);
#9384=EDGE_CURVE('',#7490,#7491,#1130,.T.);
#9385=EDGE_CURVE('',#7492,#7492,#1131,.T.);
#9386=EDGE_CURVE('',#7492,#7493,#1132,.T.);
#9387=EDGE_CURVE('',#7493,#7493,#1133,.T.);
#9388=EDGE_CURVE('',#7494,#7494,#1134,.T.);
#9389=EDGE_CURVE('',#7494,#7495,#1135,.T.);
#9390=EDGE_CURVE('',#7495,#7495,#1136,.T.);
#9391=EDGE_CURVE('',#7496,#7496,#1137,.T.);
#9392=EDGE_CURVE('',#7496,#7497,#1138,.T.);
#9393=EDGE_CURVE('',#7497,#7497,#1139,.T.);
#9394=EDGE_CURVE('',#7498,#7498,#1140,.T.);
#9395=EDGE_CURVE('',#7498,#7499,#1141,.T.);
#9396=EDGE_CURVE('',#7499,#7499,#1142,.T.);
#9397=EDGE_CURVE('',#7481,#7492,#4138,.T.);
#9398=EDGE_CURVE('',#7495,#7500,#4139,.T.);
#9399=EDGE_CURVE('',#7501,#7500,#1143,.T.);
#9400=EDGE_CURVE('',#7502,#7501,#240,.T.);
#9401=EDGE_CURVE('',#7503,#7502,#241,.T.);
#9402=EDGE_CURVE('',#7503,#7504,#1144,.T.);
#9403=EDGE_CURVE('',#7468,#7504,#242,.T.);
#9404=EDGE_CURVE('',#7459,#7467,#1145,.T.);
#9405=EDGE_CURVE('',#7505,#7461,#243,.T.);
#9406=EDGE_CURVE('',#7505,#7506,#1146,.T.);
#9407=EDGE_CURVE('',#7507,#7506,#244,.T.);
#9408=EDGE_CURVE('',#7508,#7507,#245,.T.);
#9409=EDGE_CURVE('',#7509,#7508,#1147,.T.);
#9410=EDGE_CURVE('',#7510,#7509,#246,.T.);
#9411=EDGE_CURVE('',#7511,#7510,#247,.T.);
#9412=EDGE_CURVE('',#7511,#7512,#1148,.T.);
#9413=EDGE_CURVE('',#7451,#7512,#248,.T.);
#9414=EDGE_CURVE('',#7513,#7454,#1149,.T.);
#9415=EDGE_CURVE('',#7514,#7513,#249,.T.);
#9416=EDGE_CURVE('',#7515,#7514,#250,.T.);
#9417=EDGE_CURVE('',#7515,#7516,#1150,.T.);
#9418=EDGE_CURVE('',#7517,#7516,#251,.T.);
#9419=EDGE_CURVE('',#7518,#7517,#252,.T.);
#9420=EDGE_CURVE('',#7471,#7518,#1151,.T.);
#9421=EDGE_CURVE('',#7519,#7469,#253,.T.);
#9422=EDGE_CURVE('',#7519,#7520,#1152,.T.);
#9423=EDGE_CURVE('',#7521,#7520,#254,.T.);
#9424=EDGE_CURVE('',#7522,#7521,#255,.T.);
#9425=EDGE_CURVE('',#7500,#7522,#1153,.T.);
#9426=EDGE_CURVE('',#7523,#7524,#1154,.T.);
#9427=EDGE_CURVE('',#7506,#7524,#256,.T.);
#9428=EDGE_CURVE('',#7525,#7505,#257,.T.);
#9429=EDGE_CURVE('',#7525,#7526,#1155,.T.);
#9430=EDGE_CURVE('',#7504,#7526,#258,.T.);
#9431=EDGE_CURVE('',#7527,#7503,#259,.T.);
#9432=EDGE_CURVE('',#7527,#7528,#1156,.T.);
#9433=EDGE_CURVE('',#7528,#7529,#1157,.T.);
#9434=EDGE_CURVE('',#7529,#7496,#4140,.T.);
#9435=EDGE_CURVE('',#7529,#7530,#1158,.T.);
#9436=EDGE_CURVE('',#7520,#7530,#260,.T.);
#9437=EDGE_CURVE('',#7531,#7519,#261,.T.);
#9438=EDGE_CURVE('',#7531,#7532,#1159,.T.);
#9439=EDGE_CURVE('',#7516,#7532,#262,.T.);
#9440=EDGE_CURVE('',#7533,#7515,#263,.T.);
#9441=EDGE_CURVE('',#7533,#7534,#1160,.T.);
#9442=EDGE_CURVE('',#7512,#7534,#264,.T.);
#9443=EDGE_CURVE('',#7523,#7511,#265,.T.);
#9444=EDGE_CURVE('',#7499,#7479,#4141,.T.);
#9445=EDGE_CURVE('',#7488,#7491,#4142,.T.);
#9446=EDGE_CURVE('',#7535,#7535,#1161,.T.);
#9447=EDGE_CURVE('',#7535,#7484,#4143,.T.);
#9448=EDGE_CURVE('',#7483,#7486,#4144,.T.);
#9449=EDGE_CURVE('',#7536,#7537,#1162,.T.);
#9450=EDGE_CURVE('',#7537,#7536,#1163,.T.);
#9451=EDGE_CURVE('',#7537,#7538,#1164,.T.);
#9452=EDGE_CURVE('',#7538,#7538,#1165,.T.);
#9453=EDGE_CURVE('',#7539,#7539,#1166,.T.);
#9454=EDGE_CURVE('',#7539,#7540,#1167,.T.);
#9455=EDGE_CURVE('',#7540,#7540,#1168,.T.);
#9456=EDGE_CURVE('',#7541,#7542,#1169,.T.);
#9457=EDGE_CURVE('',#7542,#7541,#1170,.T.);
#9458=EDGE_CURVE('',#7542,#7543,#1171,.T.);
#9459=EDGE_CURVE('',#7543,#7543,#1172,.T.);
#9460=EDGE_CURVE('',#7544,#7477,#4145,.T.);
#9461=EDGE_CURVE('',#7544,#7545,#1173,.T.);
#9462=EDGE_CURVE('',#7478,#7545,#4146,.T.);
#9463=EDGE_CURVE('',#7521,#7545,#1174,.T.);
#9464=EDGE_CURVE('',#7544,#7522,#1175,.T.);
#9465=EDGE_CURVE('',#7546,#7544,#1176,.T.);
#9466=EDGE_CURVE('',#7546,#7501,#1177,.T.);
#9467=EDGE_CURVE('',#7547,#7530,#4147,.T.);
#9468=EDGE_CURVE('',#7547,#7548,#266,.T.);
#9469=EDGE_CURVE('',#7549,#7548,#4148,.T.);
#9470=EDGE_CURVE('',#7545,#7549,#4149,.T.);
#9471=EDGE_CURVE('',#7550,#7551,#267,.T.);
#9472=EDGE_CURVE('',#7476,#7551,#4150,.T.);
#9473=EDGE_CURVE('',#7552,#7478,#4151,.T.);
#9474=EDGE_CURVE('',#7550,#7552,#1178,.T.);
#9475=EDGE_CURVE('',#7477,#7475,#1179,.T.);
#9476=EDGE_CURVE('',#7473,#7476,#1180,.T.);
#9477=EDGE_CURVE('',#7553,#7502,#1181,.T.);
#9478=EDGE_CURVE('',#7546,#7553,#1182,.T.);
#9479=EDGE_CURVE('',#7554,#7555,#268,.T.);
#9480=EDGE_CURVE('',#7548,#7555,#1183,.T.);
#9481=EDGE_CURVE('',#7554,#7547,#1184,.T.);
#9482=EDGE_CURVE('',#7556,#7557,#269,.T.);
#9483=EDGE_CURVE('',#7551,#7557,#1185,.T.);
#9484=EDGE_CURVE('',#7556,#7550,#1186,.T.);
#9485=EDGE_CURVE('',#7553,#7474,#4152,.T.);
#9486=EDGE_CURVE('',#7475,#7546,#4153,.T.);
#9487=EDGE_CURVE('',#7558,#7553,#4154,.T.);
#9488=EDGE_CURVE('',#7559,#7558,#4155,.T.);
#9489=EDGE_CURVE('',#7559,#7560,#270,.T.);
#9490=EDGE_CURVE('',#7527,#7560,#4156,.T.);
#9491=EDGE_CURVE('',#7531,#7554,#4157,.T.);
#9492=EDGE_CURVE('',#7561,#7470,#4158,.T.);
#9493=EDGE_CURVE('',#7555,#7561,#4159,.T.);
#9494=EDGE_CURVE('',#7562,#7563,#1187,.T.);
#9495=EDGE_CURVE('',#7557,#7563,#4160,.T.);
#9496=EDGE_CURVE('',#7564,#7556,#1188,.T.);
#9497=EDGE_CURVE('',#7562,#7564,#4161,.T.);
#9498=EDGE_CURVE('',#7565,#7566,#1189,.T.);
#9499=EDGE_CURVE('',#7474,#7565,#4162,.T.);
#9500=EDGE_CURVE('',#7567,#7473,#4163,.T.);
#9501=EDGE_CURVE('',#7567,#7566,#271,.T.);
#9502=EDGE_CURVE('',#7568,#7569,#272,.T.);
#9503=EDGE_CURVE('',#7560,#7569,#1190,.T.);
#9504=EDGE_CURVE('',#7568,#7559,#1191,.T.);
#9505=EDGE_CURVE('',#7570,#7563,#1192,.T.);
#9506=EDGE_CURVE('',#7562,#7570,#1193,.T.);
#9507=EDGE_CURVE('',#7566,#7571,#1194,.T.);
#9508=EDGE_CURVE('',#7572,#7567,#1195,.T.);
#9509=EDGE_CURVE('',#7572,#7571,#273,.T.);
#9510=EDGE_CURVE('',#7569,#7526,#4164,.T.);
#9511=EDGE_CURVE('',#7573,#7568,#4165,.T.);
#9512=EDGE_CURVE('',#7465,#7573,#4166,.T.);
#9513=EDGE_CURVE('',#7518,#7574,#1196,.T.);
#9514=EDGE_CURVE('',#7472,#7574,#1197,.T.);
#9515=EDGE_CURVE('',#7570,#7472,#4167,.T.);
#9516=EDGE_CURVE('',#7470,#7562,#4168,.T.);
#9517=EDGE_CURVE('',#7563,#7463,#1198,.T.);
#9518=EDGE_CURVE('',#7462,#7570,#1199,.T.);
#9519=EDGE_CURVE('',#7575,#7576,#1200,.T.);
#9520=EDGE_CURVE('',#7577,#7576,#4169,.T.);
#9521=EDGE_CURVE('',#7571,#7577,#1201,.T.);
#9522=EDGE_CURVE('',#7575,#7572,#4170,.T.);
#9523=EDGE_CURVE('',#7517,#7578,#1202,.T.);
#9524=EDGE_CURVE('',#7578,#7574,#1203,.T.);
#9525=EDGE_CURVE('',#7579,#7576,#1204,.T.);
#9526=EDGE_CURVE('',#7575,#7579,#1205,.T.);
#9527=EDGE_CURVE('',#7466,#7579,#4171,.T.);
#9528=EDGE_CURVE('',#7576,#7465,#4172,.T.);
#9529=EDGE_CURVE('',#7458,#7466,#1206,.T.);
#9530=EDGE_CURVE('',#7580,#7532,#4173,.T.);
#9531=EDGE_CURVE('',#7580,#7581,#274,.T.);
#9532=EDGE_CURVE('',#7582,#7581,#4174,.T.);
#9533=EDGE_CURVE('',#7578,#7582,#4175,.T.);
#9534=EDGE_CURVE('',#7464,#7578,#4176,.T.);
#9535=EDGE_CURVE('',#7574,#7462,#4177,.T.);
#9536=EDGE_CURVE('',#7583,#7584,#275,.T.);
#9537=EDGE_CURVE('',#7463,#7584,#4178,.T.);
#9538=EDGE_CURVE('',#7585,#7464,#4179,.T.);
#9539=EDGE_CURVE('',#7583,#7585,#1207,.T.);
#9540=EDGE_CURVE('',#7586,#7587,#1208,.T.);
#9541=EDGE_CURVE('',#7579,#7587,#1209,.T.);
#9542=EDGE_CURVE('',#7586,#7575,#1210,.T.);
#9543=EDGE_CURVE('',#7588,#7589,#276,.T.);
#9544=EDGE_CURVE('',#7581,#7589,#1211,.T.);
#9545=EDGE_CURVE('',#7588,#7580,#1212,.T.);
#9546=EDGE_CURVE('',#7590,#7591,#277,.T.);
#9547=EDGE_CURVE('',#7584,#7591,#1213,.T.);
#9548=EDGE_CURVE('',#7590,#7583,#1214,.T.);
#9549=EDGE_CURVE('',#7586,#7592,#1215,.T.);
#9550=EDGE_CURVE('',#7592,#7587,#1216,.T.);
#9551=EDGE_CURVE('',#7460,#7592,#4180,.T.);
#9552=EDGE_CURVE('',#7587,#7458,#4181,.T.);
#9553=EDGE_CURVE('',#7593,#7460,#4182,.T.);
#9554=EDGE_CURVE('',#7594,#7593,#4183,.T.);
#9555=EDGE_CURVE('',#7594,#7595,#278,.T.);
#9556=EDGE_CURVE('',#7525,#7595,#4184,.T.);
#9557=EDGE_CURVE('',#7533,#7588,#4185,.T.);
#9558=EDGE_CURVE('',#7514,#7596,#1217,.T.);
#9559=EDGE_CURVE('',#7597,#7596,#4186,.T.);
#9560=EDGE_CURVE('',#7589,#7597,#4187,.T.);
#9561=EDGE_CURVE('',#7591,#7457,#4188,.T.);
#9562=EDGE_CURVE('',#7598,#7590,#1218,.T.);
#9563=EDGE_CURVE('',#7455,#7598,#4189,.T.);
#9564=EDGE_CURVE('',#7599,#7600,#1219,.T.);
#9565=EDGE_CURVE('',#7592,#7599,#4190,.T.);
#9566=EDGE_CURVE('',#7601,#7586,#4191,.T.);
#9567=EDGE_CURVE('',#7601,#7600,#279,.T.);
#9568=EDGE_CURVE('',#7602,#7603,#280,.T.);
#9569=EDGE_CURVE('',#7595,#7603,#1220,.T.);
#9570=EDGE_CURVE('',#7602,#7594,#1221,.T.);
#9571=EDGE_CURVE('',#7513,#7604,#1222,.T.);
#9572=EDGE_CURVE('',#7604,#7596,#1223,.T.);
#9573=EDGE_CURVE('',#7600,#7605,#1224,.T.);
#9574=EDGE_CURVE('',#7606,#7601,#1225,.T.);
#9575=EDGE_CURVE('',#7606,#7605,#281,.T.);
#9576=EDGE_CURVE('',#7607,#7507,#1226,.T.);
#9577=EDGE_CURVE('',#7603,#7524,#4192,.T.);
#9578=EDGE_CURVE('',#7608,#7602,#4193,.T.);
#9579=EDGE_CURVE('',#7607,#7608,#4194,.T.);
#9580=EDGE_CURVE('',#7604,#7453,#1227,.T.);
#9581=EDGE_CURVE('',#7456,#7604,#4195,.T.);
#9582=EDGE_CURVE('',#7596,#7455,#4196,.T.);
#9583=EDGE_CURVE('',#7609,#7610,#1228,.T.);
#9584=EDGE_CURVE('',#7457,#7610,#1229,.T.);
#9585=EDGE_CURVE('',#7609,#7456,#1230,.T.);
#9586=EDGE_CURVE('',#7611,#7449,#4197,.T.);
#9587=EDGE_CURVE('',#7605,#7611,#1231,.T.);
#9588=EDGE_CURVE('',#7448,#7606,#4198,.T.);
#9589=EDGE_CURVE('',#7612,#7508,#1232,.T.);
#9590=EDGE_CURVE('',#7607,#7612,#1233,.T.);
#9591=EDGE_CURVE('',#7613,#7610,#1234,.T.);
#9592=EDGE_CURVE('',#7609,#7613,#1235,.T.);
#9593=EDGE_CURVE('',#7612,#7450,#4199,.T.);
#9594=EDGE_CURVE('',#7449,#7607,#4200,.T.);
#9595=EDGE_CURVE('',#7614,#7612,#1236,.T.);
#9596=EDGE_CURVE('',#7614,#7509,#1237,.T.);
#9597=EDGE_CURVE('',#7615,#7534,#4201,.T.);
#9598=EDGE_CURVE('',#7615,#7616,#282,.T.);
#9599=EDGE_CURVE('',#7617,#7616,#4202,.T.);
#9600=EDGE_CURVE('',#7452,#7617,#4203,.T.);
#9601=EDGE_CURVE('',#7613,#7452,#4204,.T.);
#9602=EDGE_CURVE('',#7453,#7609,#4205,.T.);
#9603=EDGE_CURVE('',#7618,#7619,#283,.T.);
#9604=EDGE_CURVE('',#7610,#7619,#4206,.T.);
#9605=EDGE_CURVE('',#7620,#7613,#4207,.T.);
#9606=EDGE_CURVE('',#7618,#7620,#1238,.T.);
#9607=EDGE_CURVE('',#7450,#7446,#1239,.T.);
#9608=EDGE_CURVE('',#7621,#7448,#1240,.T.);
#9609=EDGE_CURVE('',#7447,#7621,#1241,.T.);
#9610=EDGE_CURVE('',#7614,#7622,#1242,.T.);
#9611=EDGE_CURVE('',#7622,#7510,#1243,.T.);
#9612=EDGE_CURVE('',#7623,#7624,#284,.T.);
#9613=EDGE_CURVE('',#7616,#7624,#1244,.T.);
#9614=EDGE_CURVE('',#7623,#7615,#1245,.T.);
#9615=EDGE_CURVE('',#7625,#7626,#285,.T.);
#9616=EDGE_CURVE('',#7619,#7626,#1246,.T.);
#9617=EDGE_CURVE('',#7625,#7618,#1247,.T.);
#9618=EDGE_CURVE('',#7622,#7445,#4208,.T.);
#9619=EDGE_CURVE('',#7446,#7614,#4209,.T.);
#9620=EDGE_CURVE('',#7523,#7623,#4210,.T.);
#9621=EDGE_CURVE('',#7627,#7622,#4211,.T.);
#9622=EDGE_CURVE('',#7624,#7627,#4212,.T.);
#9623=EDGE_CURVE('',#7628,#7625,#1248,.T.);
#9624=EDGE_CURVE('',#7445,#7628,#4213,.T.);
#9625=EDGE_CURVE('',#7626,#7447,#4214,.T.);
#9626=EDGE_CURVE('',#7629,#7629,#1249,.T.);
#9627=EDGE_CURVE('',#7629,#7630,#1250,.T.);
#9628=EDGE_CURVE('',#7630,#7630,#1251,.T.);
#9629=EDGE_CURVE('',#7585,#7582,#4215,.T.);
#9630=EDGE_CURVE('',#7597,#7598,#4216,.T.);
#9631=EDGE_CURVE('',#7620,#7617,#4217,.T.);
#9632=EDGE_CURVE('',#7627,#7628,#4218,.T.);
#9633=EDGE_CURVE('',#7611,#7608,#4219,.T.);
#9634=EDGE_CURVE('',#7593,#7599,#4220,.T.);
#9635=EDGE_CURVE('',#7577,#7573,#4221,.T.);
#9636=EDGE_CURVE('',#7558,#7565,#4222,.T.);
#9637=EDGE_CURVE('',#7552,#7549,#4223,.T.);
#9638=EDGE_CURVE('',#7561,#7564,#4224,.T.);
#9639=EDGE_CURVE('',#7631,#7631,#1252,.T.);
#9640=EDGE_CURVE('',#7632,#7632,#1253,.T.);
#9641=EDGE_CURVE('',#7632,#7631,#1254,.T.);
#9642=EDGE_CURVE('',#7541,#7632,#4225,.T.);
#9643=EDGE_CURVE('',#7543,#7528,#4226,.T.);
#9644=EDGE_CURVE('',#7540,#7621,#4227,.T.);
#9645=EDGE_CURVE('',#7536,#7629,#4228,.T.);
#12562=ORIENTED_EDGE('',*,*,#9333,.T.);
#12563=ORIENTED_EDGE('',*,*,#9334,.F.);
#12564=ORIENTED_EDGE('',*,*,#9335,.T.);
#12565=ORIENTED_EDGE('',*,*,#9336,.F.);
#12566=ORIENTED_EDGE('',*,*,#9337,.T.);
#12567=ORIENTED_EDGE('',*,*,#9338,.T.);
#12568=ORIENTED_EDGE('',*,*,#9339,.T.);
#12569=ORIENTED_EDGE('',*,*,#9340,.T.);
#12570=ORIENTED_EDGE('',*,*,#9341,.F.);
#12571=ORIENTED_EDGE('',*,*,#9342,.T.);
#12572=ORIENTED_EDGE('',*,*,#9343,.T.);
#12573=ORIENTED_EDGE('',*,*,#9344,.T.);
#12574=ORIENTED_EDGE('',*,*,#9345,.F.);
#12575=ORIENTED_EDGE('',*,*,#9346,.F.);
#12576=ORIENTED_EDGE('',*,*,#9347,.T.);
#12577=ORIENTED_EDGE('',*,*,#9348,.T.);
#12578=ORIENTED_EDGE('',*,*,#9349,.T.);
#12579=ORIENTED_EDGE('',*,*,#9350,.F.);
#12580=ORIENTED_EDGE('',*,*,#9351,.T.);
#12581=ORIENTED_EDGE('',*,*,#9352,.T.);
#12582=ORIENTED_EDGE('',*,*,#9353,.T.);
#12583=ORIENTED_EDGE('',*,*,#9354,.T.);
#12584=ORIENTED_EDGE('',*,*,#9355,.T.);
#12585=ORIENTED_EDGE('',*,*,#9356,.F.);
#12586=ORIENTED_EDGE('',*,*,#9357,.F.);
#12587=ORIENTED_EDGE('',*,*,#9358,.T.);
#12588=ORIENTED_EDGE('',*,*,#9359,.T.);
#12589=ORIENTED_EDGE('',*,*,#9360,.T.);
#12590=ORIENTED_EDGE('',*,*,#9361,.T.);
#12591=ORIENTED_EDGE('',*,*,#9362,.T.);
#12592=ORIENTED_EDGE('',*,*,#9363,.F.);
#12593=ORIENTED_EDGE('',*,*,#9364,.T.);
#12594=ORIENTED_EDGE('',*,*,#9365,.F.);
#12595=ORIENTED_EDGE('',*,*,#9366,.T.);
#12596=ORIENTED_EDGE('',*,*,#9367,.F.);
#12597=ORIENTED_EDGE('',*,*,#9368,.T.);
#12598=ORIENTED_EDGE('',*,*,#9369,.F.);
#12599=ORIENTED_EDGE('',*,*,#9368,.F.);
#12600=ORIENTED_EDGE('',*,*,#9370,.F.);
#12601=ORIENTED_EDGE('',*,*,#9371,.F.);
#12602=ORIENTED_EDGE('',*,*,#9372,.T.);
#12603=ORIENTED_EDGE('',*,*,#9373,.F.);
#12604=ORIENTED_EDGE('',*,*,#9372,.F.);
#12605=ORIENTED_EDGE('',*,*,#9374,.F.);
#12606=ORIENTED_EDGE('',*,*,#9375,.T.);
#12607=ORIENTED_EDGE('',*,*,#9376,.F.);
#12608=ORIENTED_EDGE('',*,*,#9377,.F.);
#12609=ORIENTED_EDGE('',*,*,#9375,.F.);
#12610=ORIENTED_EDGE('',*,*,#9378,.F.);
#12611=ORIENTED_EDGE('',*,*,#9379,.T.);
#12612=ORIENTED_EDGE('',*,*,#9380,.F.);
#12613=ORIENTED_EDGE('',*,*,#9379,.F.);
#12614=ORIENTED_EDGE('',*,*,#9381,.F.);
#12615=ORIENTED_EDGE('',*,*,#9382,.T.);
#12616=ORIENTED_EDGE('',*,*,#9383,.F.);
#12617=ORIENTED_EDGE('',*,*,#9384,.F.);
#12618=ORIENTED_EDGE('',*,*,#9382,.F.);
#12619=ORIENTED_EDGE('',*,*,#9385,.F.);
#12620=ORIENTED_EDGE('',*,*,#9386,.T.);
#12621=ORIENTED_EDGE('',*,*,#9387,.F.);
#12622=ORIENTED_EDGE('',*,*,#9386,.F.);
#12623=ORIENTED_EDGE('',*,*,#9388,.F.);
#12624=ORIENTED_EDGE('',*,*,#9389,.T.);
#12625=ORIENTED_EDGE('',*,*,#9390,.F.);
#12626=ORIENTED_EDGE('',*,*,#9389,.F.);
#12627=ORIENTED_EDGE('',*,*,#9391,.F.);
#12628=ORIENTED_EDGE('',*,*,#9392,.T.);
#12629=ORIENTED_EDGE('',*,*,#9393,.F.);
#12630=ORIENTED_EDGE('',*,*,#9392,.F.);
#12631=ORIENTED_EDGE('',*,*,#9394,.F.);
#12632=ORIENTED_EDGE('',*,*,#9395,.T.);
#12633=ORIENTED_EDGE('',*,*,#9396,.F.);
#12634=ORIENTED_EDGE('',*,*,#9395,.F.);
#12635=ORIENTED_EDGE('',*,*,#9370,.T.);
#12636=ORIENTED_EDGE('',*,*,#9371,.T.);
#12637=ORIENTED_EDGE('',*,*,#9397,.T.);
#12638=ORIENTED_EDGE('',*,*,#9385,.T.);
#12639=ORIENTED_EDGE('',*,*,#9397,.F.);
#12640=ORIENTED_EDGE('',*,*,#9390,.T.);
#12641=ORIENTED_EDGE('',*,*,#9398,.T.);
#12642=ORIENTED_EDGE('',*,*,#9399,.F.);
#12643=ORIENTED_EDGE('',*,*,#9400,.F.);
#12644=ORIENTED_EDGE('',*,*,#9401,.F.);
#12645=ORIENTED_EDGE('',*,*,#9402,.T.);
#12646=ORIENTED_EDGE('',*,*,#9403,.F.);
#12647=ORIENTED_EDGE('',*,*,#9355,.F.);
#12648=ORIENTED_EDGE('',*,*,#9404,.F.);
#12649=ORIENTED_EDGE('',*,*,#9349,.F.);
#12650=ORIENTED_EDGE('',*,*,#9405,.F.);
#12651=ORIENTED_EDGE('',*,*,#9406,.T.);
#12652=ORIENTED_EDGE('',*,*,#9407,.F.);
#12653=ORIENTED_EDGE('',*,*,#9408,.F.);
#12654=ORIENTED_EDGE('',*,*,#9409,.F.);
#12655=ORIENTED_EDGE('',*,*,#9410,.F.);
#12656=ORIENTED_EDGE('',*,*,#9411,.F.);
#12657=ORIENTED_EDGE('',*,*,#9412,.T.);
#12658=ORIENTED_EDGE('',*,*,#9413,.F.);
#12659=ORIENTED_EDGE('',*,*,#9342,.F.);
#12660=ORIENTED_EDGE('',*,*,#9414,.F.);
#12661=ORIENTED_EDGE('',*,*,#9415,.F.);
#12662=ORIENTED_EDGE('',*,*,#9416,.F.);
#12663=ORIENTED_EDGE('',*,*,#9417,.T.);
#12664=ORIENTED_EDGE('',*,*,#9418,.F.);
#12665=ORIENTED_EDGE('',*,*,#9419,.F.);
#12666=ORIENTED_EDGE('',*,*,#9420,.F.);
#12667=ORIENTED_EDGE('',*,*,#9358,.F.);
#12668=ORIENTED_EDGE('',*,*,#9421,.F.);
#12669=ORIENTED_EDGE('',*,*,#9422,.T.);
#12670=ORIENTED_EDGE('',*,*,#9423,.F.);
#12671=ORIENTED_EDGE('',*,*,#9424,.F.);
#12672=ORIENTED_EDGE('',*,*,#9425,.F.);
#12673=ORIENTED_EDGE('',*,*,#9398,.F.);
#12674=ORIENTED_EDGE('',*,*,#9426,.T.);
#12675=ORIENTED_EDGE('',*,*,#9427,.F.);
#12676=ORIENTED_EDGE('',*,*,#9406,.F.);
#12677=ORIENTED_EDGE('',*,*,#9428,.F.);
#12678=ORIENTED_EDGE('',*,*,#9429,.T.);
#12679=ORIENTED_EDGE('',*,*,#9430,.F.);
#12680=ORIENTED_EDGE('',*,*,#9402,.F.);
#12681=ORIENTED_EDGE('',*,*,#9431,.F.);
#12682=ORIENTED_EDGE('',*,*,#9432,.T.);
#12683=ORIENTED_EDGE('',*,*,#9433,.T.);
#12684=ORIENTED_EDGE('',*,*,#9434,.T.);
#12685=ORIENTED_EDGE('',*,*,#9391,.T.);
#12686=ORIENTED_EDGE('',*,*,#9434,.F.);
#12687=ORIENTED_EDGE('',*,*,#9435,.T.);
#12688=ORIENTED_EDGE('',*,*,#9436,.F.);
#12689=ORIENTED_EDGE('',*,*,#9422,.F.);
#12690=ORIENTED_EDGE('',*,*,#9437,.F.);
#12691=ORIENTED_EDGE('',*,*,#9438,.T.);
#12692=ORIENTED_EDGE('',*,*,#9439,.F.);
#12693=ORIENTED_EDGE('',*,*,#9417,.F.);
#12694=ORIENTED_EDGE('',*,*,#9440,.F.);
#12695=ORIENTED_EDGE('',*,*,#9441,.T.);
#12696=ORIENTED_EDGE('',*,*,#9442,.F.);
#12697=ORIENTED_EDGE('',*,*,#9412,.F.);
#12698=ORIENTED_EDGE('',*,*,#9443,.F.);
#12699=ORIENTED_EDGE('',*,*,#9393,.T.);
#12700=ORIENTED_EDGE('',*,*,#9394,.T.);
#12701=ORIENTED_EDGE('',*,*,#9396,.T.);
#12702=ORIENTED_EDGE('',*,*,#9444,.T.);
#12703=ORIENTED_EDGE('',*,*,#9367,.T.);
#12704=ORIENTED_EDGE('',*,*,#9444,.F.);
#12705=ORIENTED_EDGE('',*,*,#9369,.T.);
#12706=ORIENTED_EDGE('',*,*,#9378,.T.);
#12707=ORIENTED_EDGE('',*,*,#9380,.T.);
#12708=ORIENTED_EDGE('',*,*,#9445,.T.);
#12709=ORIENTED_EDGE('',*,*,#9383,.T.);
#12710=ORIENTED_EDGE('',*,*,#9384,.T.);
#12711=ORIENTED_EDGE('',*,*,#9445,.F.);
#12712=ORIENTED_EDGE('',*,*,#9446,.T.);
#12713=ORIENTED_EDGE('',*,*,#9381,.T.);
#12714=ORIENTED_EDGE('',*,*,#9446,.F.);
#12715=ORIENTED_EDGE('',*,*,#9447,.T.);
#12716=ORIENTED_EDGE('',*,*,#9374,.T.);
#12717=ORIENTED_EDGE('',*,*,#9447,.F.);
#12718=ORIENTED_EDGE('',*,*,#9373,.T.);
#12719=ORIENTED_EDGE('',*,*,#9448,.T.);
#12720=ORIENTED_EDGE('',*,*,#9376,.T.);
#12721=ORIENTED_EDGE('',*,*,#9377,.T.);
#12722=ORIENTED_EDGE('',*,*,#9448,.F.);
#12723=ORIENTED_EDGE('',*,*,#9387,.T.);
#12724=ORIENTED_EDGE('',*,*,#9388,.T.);
#12725=ORIENTED_EDGE('',*,*,#9449,.F.);
#12726=ORIENTED_EDGE('',*,*,#9450,.F.);
#12727=ORIENTED_EDGE('',*,*,#9451,.T.);
#12728=ORIENTED_EDGE('',*,*,#9452,.F.);
#12729=ORIENTED_EDGE('',*,*,#9451,.F.);
#12730=ORIENTED_EDGE('',*,*,#9453,.F.);
#12731=ORIENTED_EDGE('',*,*,#9454,.T.);
#12732=ORIENTED_EDGE('',*,*,#9455,.F.);
#12733=ORIENTED_EDGE('',*,*,#9454,.F.);
#12734=ORIENTED_EDGE('',*,*,#9456,.F.);
#12735=ORIENTED_EDGE('',*,*,#9457,.F.);
#12736=ORIENTED_EDGE('',*,*,#9458,.T.);
#12737=ORIENTED_EDGE('',*,*,#9459,.F.);
#12738=ORIENTED_EDGE('',*,*,#9458,.F.);
#12739=ORIENTED_EDGE('',*,*,#9365,.T.);
#12740=ORIENTED_EDGE('',*,*,#9460,.F.);
#12741=ORIENTED_EDGE('',*,*,#9461,.T.);
#12742=ORIENTED_EDGE('',*,*,#9462,.F.);
#12743=ORIENTED_EDGE('',*,*,#9463,.T.);
#12744=ORIENTED_EDGE('',*,*,#9461,.F.);
#12745=ORIENTED_EDGE('',*,*,#9464,.T.);
#12746=ORIENTED_EDGE('',*,*,#9424,.T.);
#12747=ORIENTED_EDGE('',*,*,#9399,.T.);
#12748=ORIENTED_EDGE('',*,*,#9425,.T.);
#12749=ORIENTED_EDGE('',*,*,#9464,.F.);
#12750=ORIENTED_EDGE('',*,*,#9465,.F.);
#12751=ORIENTED_EDGE('',*,*,#9466,.T.);
#12752=ORIENTED_EDGE('',*,*,#9423,.T.);
#12753=ORIENTED_EDGE('',*,*,#9436,.T.);
#12754=ORIENTED_EDGE('',*,*,#9467,.F.);
#12755=ORIENTED_EDGE('',*,*,#9468,.T.);
#12756=ORIENTED_EDGE('',*,*,#9469,.F.);
#12757=ORIENTED_EDGE('',*,*,#9470,.F.);
#12758=ORIENTED_EDGE('',*,*,#9463,.F.);
#12759=ORIENTED_EDGE('',*,*,#9471,.T.);
#12760=ORIENTED_EDGE('',*,*,#9472,.F.);
#12761=ORIENTED_EDGE('',*,*,#9366,.F.);
#12762=ORIENTED_EDGE('',*,*,#9473,.F.);
#12763=ORIENTED_EDGE('',*,*,#9474,.F.);
#12764=ORIENTED_EDGE('',*,*,#9475,.F.);
#12765=ORIENTED_EDGE('',*,*,#9364,.F.);
#12766=ORIENTED_EDGE('',*,*,#9476,.F.);
#12767=ORIENTED_EDGE('',*,*,#9363,.T.);
#12768=ORIENTED_EDGE('',*,*,#9477,.T.);
#12769=ORIENTED_EDGE('',*,*,#9400,.T.);
#12770=ORIENTED_EDGE('',*,*,#9466,.F.);
#12771=ORIENTED_EDGE('',*,*,#9478,.T.);
#12772=ORIENTED_EDGE('',*,*,#9479,.T.);
#12773=ORIENTED_EDGE('',*,*,#9480,.F.);
#12774=ORIENTED_EDGE('',*,*,#9468,.F.);
#12775=ORIENTED_EDGE('',*,*,#9481,.F.);
#12776=ORIENTED_EDGE('',*,*,#9482,.T.);
#12777=ORIENTED_EDGE('',*,*,#9483,.F.);
#12778=ORIENTED_EDGE('',*,*,#9471,.F.);
#12779=ORIENTED_EDGE('',*,*,#9484,.F.);
#12780=ORIENTED_EDGE('',*,*,#9362,.F.);
#12781=ORIENTED_EDGE('',*,*,#9485,.F.);
#12782=ORIENTED_EDGE('',*,*,#9478,.F.);
#12783=ORIENTED_EDGE('',*,*,#9486,.F.);
#12784=ORIENTED_EDGE('',*,*,#9431,.T.);
#12785=ORIENTED_EDGE('',*,*,#9401,.T.);
#12786=ORIENTED_EDGE('',*,*,#9477,.F.);
#12787=ORIENTED_EDGE('',*,*,#9487,.F.);
#12788=ORIENTED_EDGE('',*,*,#9488,.F.);
#12789=ORIENTED_EDGE('',*,*,#9489,.T.);
#12790=ORIENTED_EDGE('',*,*,#9490,.F.);
#12791=ORIENTED_EDGE('',*,*,#9491,.F.);
#12792=ORIENTED_EDGE('',*,*,#9437,.T.);
#12793=ORIENTED_EDGE('',*,*,#9421,.T.);
#12794=ORIENTED_EDGE('',*,*,#9357,.T.);
#12795=ORIENTED_EDGE('',*,*,#9492,.F.);
#12796=ORIENTED_EDGE('',*,*,#9493,.F.);
#12797=ORIENTED_EDGE('',*,*,#9479,.F.);
#12798=ORIENTED_EDGE('',*,*,#9494,.T.);
#12799=ORIENTED_EDGE('',*,*,#9495,.F.);
#12800=ORIENTED_EDGE('',*,*,#9482,.F.);
#12801=ORIENTED_EDGE('',*,*,#9496,.F.);
#12802=ORIENTED_EDGE('',*,*,#9497,.F.);
#12803=ORIENTED_EDGE('',*,*,#9498,.F.);
#12804=ORIENTED_EDGE('',*,*,#9499,.F.);
#12805=ORIENTED_EDGE('',*,*,#9361,.F.);
#12806=ORIENTED_EDGE('',*,*,#9500,.F.);
#12807=ORIENTED_EDGE('',*,*,#9501,.T.);
#12808=ORIENTED_EDGE('',*,*,#9502,.T.);
#12809=ORIENTED_EDGE('',*,*,#9503,.F.);
#12810=ORIENTED_EDGE('',*,*,#9489,.F.);
#12811=ORIENTED_EDGE('',*,*,#9504,.F.);
#12812=ORIENTED_EDGE('',*,*,#9505,.T.);
#12813=ORIENTED_EDGE('',*,*,#9494,.F.);
#12814=ORIENTED_EDGE('',*,*,#9506,.T.);
#12815=ORIENTED_EDGE('',*,*,#9507,.F.);
#12816=ORIENTED_EDGE('',*,*,#9501,.F.);
#12817=ORIENTED_EDGE('',*,*,#9508,.F.);
#12818=ORIENTED_EDGE('',*,*,#9509,.T.);
#12819=ORIENTED_EDGE('',*,*,#9356,.T.);
#12820=ORIENTED_EDGE('',*,*,#9403,.T.);
#12821=ORIENTED_EDGE('',*,*,#9430,.T.);
#12822=ORIENTED_EDGE('',*,*,#9510,.F.);
#12823=ORIENTED_EDGE('',*,*,#9502,.F.);
#12824=ORIENTED_EDGE('',*,*,#9511,.F.);
#12825=ORIENTED_EDGE('',*,*,#9512,.F.);
#12826=ORIENTED_EDGE('',*,*,#9359,.F.);
#12827=ORIENTED_EDGE('',*,*,#9420,.T.);
#12828=ORIENTED_EDGE('',*,*,#9513,.T.);
#12829=ORIENTED_EDGE('',*,*,#9514,.F.);
#12830=ORIENTED_EDGE('',*,*,#9360,.F.);
#12831=ORIENTED_EDGE('',*,*,#9515,.F.);
#12832=ORIENTED_EDGE('',*,*,#9506,.F.);
#12833=ORIENTED_EDGE('',*,*,#9516,.F.);
#12834=ORIENTED_EDGE('',*,*,#9350,.T.);
#12835=ORIENTED_EDGE('',*,*,#9517,.F.);
#12836=ORIENTED_EDGE('',*,*,#9505,.F.);
#12837=ORIENTED_EDGE('',*,*,#9518,.F.);
#12838=ORIENTED_EDGE('',*,*,#9519,.T.);
#12839=ORIENTED_EDGE('',*,*,#9520,.F.);
#12840=ORIENTED_EDGE('',*,*,#9521,.F.);
#12841=ORIENTED_EDGE('',*,*,#9509,.F.);
#12842=ORIENTED_EDGE('',*,*,#9522,.F.);
#12843=ORIENTED_EDGE('',*,*,#9513,.F.);
#12844=ORIENTED_EDGE('',*,*,#9419,.T.);
#12845=ORIENTED_EDGE('',*,*,#9523,.T.);
#12846=ORIENTED_EDGE('',*,*,#9524,.T.);
#12847=ORIENTED_EDGE('',*,*,#9525,.T.);
#12848=ORIENTED_EDGE('',*,*,#9519,.F.);
#12849=ORIENTED_EDGE('',*,*,#9526,.T.);
#12850=ORIENTED_EDGE('',*,*,#9525,.F.);
#12851=ORIENTED_EDGE('',*,*,#9527,.F.);
#12852=ORIENTED_EDGE('',*,*,#9353,.F.);
#12853=ORIENTED_EDGE('',*,*,#9528,.F.);
#12854=ORIENTED_EDGE('',*,*,#9346,.T.);
#12855=ORIENTED_EDGE('',*,*,#9404,.T.);
#12856=ORIENTED_EDGE('',*,*,#9354,.F.);
#12857=ORIENTED_EDGE('',*,*,#9529,.F.);
#12858=ORIENTED_EDGE('',*,*,#9418,.T.);
#12859=ORIENTED_EDGE('',*,*,#9439,.T.);
#12860=ORIENTED_EDGE('',*,*,#9530,.F.);
#12861=ORIENTED_EDGE('',*,*,#9531,.T.);
#12862=ORIENTED_EDGE('',*,*,#9532,.F.);
#12863=ORIENTED_EDGE('',*,*,#9533,.F.);
#12864=ORIENTED_EDGE('',*,*,#9523,.F.);
#12865=ORIENTED_EDGE('',*,*,#9524,.F.);
#12866=ORIENTED_EDGE('',*,*,#9534,.F.);
#12867=ORIENTED_EDGE('',*,*,#9351,.F.);
#12868=ORIENTED_EDGE('',*,*,#9535,.F.);
#12869=ORIENTED_EDGE('',*,*,#9536,.T.);
#12870=ORIENTED_EDGE('',*,*,#9537,.F.);
#12871=ORIENTED_EDGE('',*,*,#9352,.F.);
#12872=ORIENTED_EDGE('',*,*,#9538,.F.);
#12873=ORIENTED_EDGE('',*,*,#9539,.F.);
#12874=ORIENTED_EDGE('',*,*,#9540,.T.);
#12875=ORIENTED_EDGE('',*,*,#9541,.F.);
#12876=ORIENTED_EDGE('',*,*,#9526,.F.);
#12877=ORIENTED_EDGE('',*,*,#9542,.F.);
#12878=ORIENTED_EDGE('',*,*,#9543,.T.);
#12879=ORIENTED_EDGE('',*,*,#9544,.F.);
#12880=ORIENTED_EDGE('',*,*,#9531,.F.);
#12881=ORIENTED_EDGE('',*,*,#9545,.F.);
#12882=ORIENTED_EDGE('',*,*,#9546,.T.);
#12883=ORIENTED_EDGE('',*,*,#9547,.F.);
#12884=ORIENTED_EDGE('',*,*,#9536,.F.);
#12885=ORIENTED_EDGE('',*,*,#9548,.F.);
#12886=ORIENTED_EDGE('',*,*,#9549,.T.);
#12887=ORIENTED_EDGE('',*,*,#9550,.T.);
#12888=ORIENTED_EDGE('',*,*,#9540,.F.);
#12889=ORIENTED_EDGE('',*,*,#9550,.F.);
#12890=ORIENTED_EDGE('',*,*,#9551,.F.);
#12891=ORIENTED_EDGE('',*,*,#9347,.F.);
#12892=ORIENTED_EDGE('',*,*,#9552,.F.);
#12893=ORIENTED_EDGE('',*,*,#9428,.T.);
#12894=ORIENTED_EDGE('',*,*,#9405,.T.);
#12895=ORIENTED_EDGE('',*,*,#9348,.F.);
#12896=ORIENTED_EDGE('',*,*,#9553,.F.);
#12897=ORIENTED_EDGE('',*,*,#9554,.F.);
#12898=ORIENTED_EDGE('',*,*,#9555,.T.);
#12899=ORIENTED_EDGE('',*,*,#9556,.F.);
#12900=ORIENTED_EDGE('',*,*,#9557,.F.);
#12901=ORIENTED_EDGE('',*,*,#9440,.T.);
#12902=ORIENTED_EDGE('',*,*,#9416,.T.);
#12903=ORIENTED_EDGE('',*,*,#9558,.T.);
#12904=ORIENTED_EDGE('',*,*,#9559,.F.);
#12905=ORIENTED_EDGE('',*,*,#9560,.F.);
#12906=ORIENTED_EDGE('',*,*,#9543,.F.);
#12907=ORIENTED_EDGE('',*,*,#9345,.T.);
#12908=ORIENTED_EDGE('',*,*,#9561,.F.);
#12909=ORIENTED_EDGE('',*,*,#9546,.F.);
#12910=ORIENTED_EDGE('',*,*,#9562,.F.);
#12911=ORIENTED_EDGE('',*,*,#9563,.F.);
#12912=ORIENTED_EDGE('',*,*,#9564,.F.);
#12913=ORIENTED_EDGE('',*,*,#9565,.F.);
#12914=ORIENTED_EDGE('',*,*,#9549,.F.);
#12915=ORIENTED_EDGE('',*,*,#9566,.F.);
#12916=ORIENTED_EDGE('',*,*,#9567,.T.);
#12917=ORIENTED_EDGE('',*,*,#9568,.T.);
#12918=ORIENTED_EDGE('',*,*,#9569,.F.);
#12919=ORIENTED_EDGE('',*,*,#9555,.F.);
#12920=ORIENTED_EDGE('',*,*,#9570,.F.);
#12921=ORIENTED_EDGE('',*,*,#9558,.F.);
#12922=ORIENTED_EDGE('',*,*,#9415,.T.);
#12923=ORIENTED_EDGE('',*,*,#9571,.T.);
#12924=ORIENTED_EDGE('',*,*,#9572,.T.);
#12925=ORIENTED_EDGE('',*,*,#9573,.F.);
#12926=ORIENTED_EDGE('',*,*,#9567,.F.);
#12927=ORIENTED_EDGE('',*,*,#9574,.F.);
#12928=ORIENTED_EDGE('',*,*,#9575,.T.);
#12929=ORIENTED_EDGE('',*,*,#9576,.T.);
#12930=ORIENTED_EDGE('',*,*,#9407,.T.);
#12931=ORIENTED_EDGE('',*,*,#9427,.T.);
#12932=ORIENTED_EDGE('',*,*,#9577,.F.);
#12933=ORIENTED_EDGE('',*,*,#9568,.F.);
#12934=ORIENTED_EDGE('',*,*,#9578,.F.);
#12935=ORIENTED_EDGE('',*,*,#9579,.F.);
#12936=ORIENTED_EDGE('',*,*,#9571,.F.);
#12937=ORIENTED_EDGE('',*,*,#9414,.T.);
#12938=ORIENTED_EDGE('',*,*,#9341,.T.);
#12939=ORIENTED_EDGE('',*,*,#9580,.F.);
#12940=ORIENTED_EDGE('',*,*,#9572,.F.);
#12941=ORIENTED_EDGE('',*,*,#9581,.F.);
#12942=ORIENTED_EDGE('',*,*,#9343,.F.);
#12943=ORIENTED_EDGE('',*,*,#9582,.F.);
#12944=ORIENTED_EDGE('',*,*,#9583,.T.);
#12945=ORIENTED_EDGE('',*,*,#9584,.F.);
#12946=ORIENTED_EDGE('',*,*,#9344,.F.);
#12947=ORIENTED_EDGE('',*,*,#9585,.F.);
#12948=ORIENTED_EDGE('',*,*,#9586,.F.);
#12949=ORIENTED_EDGE('',*,*,#9587,.F.);
#12950=ORIENTED_EDGE('',*,*,#9575,.F.);
#12951=ORIENTED_EDGE('',*,*,#9588,.F.);
#12952=ORIENTED_EDGE('',*,*,#9336,.T.);
#12953=ORIENTED_EDGE('',*,*,#9589,.T.);
#12954=ORIENTED_EDGE('',*,*,#9408,.T.);
#12955=ORIENTED_EDGE('',*,*,#9576,.F.);
#12956=ORIENTED_EDGE('',*,*,#9590,.T.);
#12957=ORIENTED_EDGE('',*,*,#9591,.T.);
#12958=ORIENTED_EDGE('',*,*,#9583,.F.);
#12959=ORIENTED_EDGE('',*,*,#9592,.T.);
#12960=ORIENTED_EDGE('',*,*,#9338,.F.);
#12961=ORIENTED_EDGE('',*,*,#9593,.F.);
#12962=ORIENTED_EDGE('',*,*,#9590,.F.);
#12963=ORIENTED_EDGE('',*,*,#9594,.F.);
#12964=ORIENTED_EDGE('',*,*,#9409,.T.);
#12965=ORIENTED_EDGE('',*,*,#9589,.F.);
#12966=ORIENTED_EDGE('',*,*,#9595,.F.);
#12967=ORIENTED_EDGE('',*,*,#9596,.T.);
#12968=ORIENTED_EDGE('',*,*,#9413,.T.);
#12969=ORIENTED_EDGE('',*,*,#9442,.T.);
#12970=ORIENTED_EDGE('',*,*,#9597,.F.);
#12971=ORIENTED_EDGE('',*,*,#9598,.T.);
#12972=ORIENTED_EDGE('',*,*,#9599,.F.);
#12973=ORIENTED_EDGE('',*,*,#9600,.F.);
#12974=ORIENTED_EDGE('',*,*,#9339,.F.);
#12975=ORIENTED_EDGE('',*,*,#9340,.F.);
#12976=ORIENTED_EDGE('',*,*,#9601,.F.);
#12977=ORIENTED_EDGE('',*,*,#9592,.F.);
#12978=ORIENTED_EDGE('',*,*,#9602,.F.);
#12979=ORIENTED_EDGE('',*,*,#9603,.T.);
#12980=ORIENTED_EDGE('',*,*,#9604,.F.);
#12981=ORIENTED_EDGE('',*,*,#9591,.F.);
#12982=ORIENTED_EDGE('',*,*,#9605,.F.);
#12983=ORIENTED_EDGE('',*,*,#9606,.F.);
#12984=ORIENTED_EDGE('',*,*,#9334,.T.);
#12985=ORIENTED_EDGE('',*,*,#9607,.F.);
#12986=ORIENTED_EDGE('',*,*,#9337,.F.);
#12987=ORIENTED_EDGE('',*,*,#9608,.F.);
#12988=ORIENTED_EDGE('',*,*,#9609,.F.);
#12989=ORIENTED_EDGE('',*,*,#9610,.T.);
#12990=ORIENTED_EDGE('',*,*,#9611,.T.);
#12991=ORIENTED_EDGE('',*,*,#9410,.T.);
#12992=ORIENTED_EDGE('',*,*,#9596,.F.);
#12993=ORIENTED_EDGE('',*,*,#9612,.T.);
#12994=ORIENTED_EDGE('',*,*,#9613,.F.);
#12995=ORIENTED_EDGE('',*,*,#9598,.F.);
#12996=ORIENTED_EDGE('',*,*,#9614,.F.);
#12997=ORIENTED_EDGE('',*,*,#9615,.T.);
#12998=ORIENTED_EDGE('',*,*,#9616,.F.);
#12999=ORIENTED_EDGE('',*,*,#9603,.F.);
#13000=ORIENTED_EDGE('',*,*,#9617,.F.);
#13001=ORIENTED_EDGE('',*,*,#9333,.F.);
#13002=ORIENTED_EDGE('',*,*,#9618,.F.);
#13003=ORIENTED_EDGE('',*,*,#9610,.F.);
#13004=ORIENTED_EDGE('',*,*,#9619,.F.);
#13005=ORIENTED_EDGE('',*,*,#9620,.F.);
#13006=ORIENTED_EDGE('',*,*,#9443,.T.);
#13007=ORIENTED_EDGE('',*,*,#9411,.T.);
#13008=ORIENTED_EDGE('',*,*,#9611,.F.);
#13009=ORIENTED_EDGE('',*,*,#9621,.F.);
#13010=ORIENTED_EDGE('',*,*,#9622,.F.);
#13011=ORIENTED_EDGE('',*,*,#9612,.F.);
#13012=ORIENTED_EDGE('',*,*,#9623,.F.);
#13013=ORIENTED_EDGE('',*,*,#9624,.F.);
#13014=ORIENTED_EDGE('',*,*,#9335,.F.);
#13015=ORIENTED_EDGE('',*,*,#9625,.F.);
#13016=ORIENTED_EDGE('',*,*,#9615,.F.);
#13017=ORIENTED_EDGE('',*,*,#9626,.F.);
#13018=ORIENTED_EDGE('',*,*,#9627,.T.);
#13019=ORIENTED_EDGE('',*,*,#9628,.F.);
#13020=ORIENTED_EDGE('',*,*,#9627,.F.);
#13021=ORIENTED_EDGE('',*,*,#9629,.T.);
#13022=ORIENTED_EDGE('',*,*,#9532,.T.);
#13023=ORIENTED_EDGE('',*,*,#9544,.T.);
#13024=ORIENTED_EDGE('',*,*,#9560,.T.);
#13025=ORIENTED_EDGE('',*,*,#9630,.T.);
#13026=ORIENTED_EDGE('',*,*,#9562,.T.);
#13027=ORIENTED_EDGE('',*,*,#9548,.T.);
#13028=ORIENTED_EDGE('',*,*,#9539,.T.);
#13029=ORIENTED_EDGE('',*,*,#9630,.F.);
#13030=ORIENTED_EDGE('',*,*,#9559,.T.);
#13031=ORIENTED_EDGE('',*,*,#9582,.T.);
#13032=ORIENTED_EDGE('',*,*,#9563,.T.);
#13033=ORIENTED_EDGE('',*,*,#9534,.T.);
#13034=ORIENTED_EDGE('',*,*,#9533,.T.);
#13035=ORIENTED_EDGE('',*,*,#9629,.F.);
#13036=ORIENTED_EDGE('',*,*,#9538,.T.);
#13037=ORIENTED_EDGE('',*,*,#9631,.T.);
#13038=ORIENTED_EDGE('',*,*,#9599,.T.);
#13039=ORIENTED_EDGE('',*,*,#9613,.T.);
#13040=ORIENTED_EDGE('',*,*,#9622,.T.);
#13041=ORIENTED_EDGE('',*,*,#9632,.T.);
#13042=ORIENTED_EDGE('',*,*,#9623,.T.);
#13043=ORIENTED_EDGE('',*,*,#9617,.T.);
#13044=ORIENTED_EDGE('',*,*,#9606,.T.);
#13045=ORIENTED_EDGE('',*,*,#9601,.T.);
#13046=ORIENTED_EDGE('',*,*,#9600,.T.);
#13047=ORIENTED_EDGE('',*,*,#9631,.F.);
#13048=ORIENTED_EDGE('',*,*,#9605,.T.);
#13049=ORIENTED_EDGE('',*,*,#9632,.F.);
#13050=ORIENTED_EDGE('',*,*,#9621,.T.);
#13051=ORIENTED_EDGE('',*,*,#9618,.T.);
#13052=ORIENTED_EDGE('',*,*,#9624,.T.);
#13053=ORIENTED_EDGE('',*,*,#9633,.T.);
#13054=ORIENTED_EDGE('',*,*,#9578,.T.);
#13055=ORIENTED_EDGE('',*,*,#9570,.T.);
#13056=ORIENTED_EDGE('',*,*,#9554,.T.);
#13057=ORIENTED_EDGE('',*,*,#9634,.T.);
#13058=ORIENTED_EDGE('',*,*,#9564,.T.);
#13059=ORIENTED_EDGE('',*,*,#9573,.T.);
#13060=ORIENTED_EDGE('',*,*,#9587,.T.);
#13061=ORIENTED_EDGE('',*,*,#9594,.T.);
#13062=ORIENTED_EDGE('',*,*,#9579,.T.);
#13063=ORIENTED_EDGE('',*,*,#9633,.F.);
#13064=ORIENTED_EDGE('',*,*,#9586,.T.);
#13065=ORIENTED_EDGE('',*,*,#9634,.F.);
#13066=ORIENTED_EDGE('',*,*,#9553,.T.);
#13067=ORIENTED_EDGE('',*,*,#9551,.T.);
#13068=ORIENTED_EDGE('',*,*,#9565,.T.);
#13069=ORIENTED_EDGE('',*,*,#9635,.T.);
#13070=ORIENTED_EDGE('',*,*,#9511,.T.);
#13071=ORIENTED_EDGE('',*,*,#9504,.T.);
#13072=ORIENTED_EDGE('',*,*,#9488,.T.);
#13073=ORIENTED_EDGE('',*,*,#9636,.T.);
#13074=ORIENTED_EDGE('',*,*,#9498,.T.);
#13075=ORIENTED_EDGE('',*,*,#9507,.T.);
#13076=ORIENTED_EDGE('',*,*,#9521,.T.);
#13077=ORIENTED_EDGE('',*,*,#9528,.T.);
#13078=ORIENTED_EDGE('',*,*,#9512,.T.);
#13079=ORIENTED_EDGE('',*,*,#9635,.F.);
#13080=ORIENTED_EDGE('',*,*,#9520,.T.);
#13081=ORIENTED_EDGE('',*,*,#9636,.F.);
#13082=ORIENTED_EDGE('',*,*,#9487,.T.);
#13083=ORIENTED_EDGE('',*,*,#9485,.T.);
#13084=ORIENTED_EDGE('',*,*,#9499,.T.);
#13085=ORIENTED_EDGE('',*,*,#9637,.T.);
#13086=ORIENTED_EDGE('',*,*,#9469,.T.);
#13087=ORIENTED_EDGE('',*,*,#9480,.T.);
#13088=ORIENTED_EDGE('',*,*,#9493,.T.);
#13089=ORIENTED_EDGE('',*,*,#9638,.T.);
#13090=ORIENTED_EDGE('',*,*,#9496,.T.);
#13091=ORIENTED_EDGE('',*,*,#9484,.T.);
#13092=ORIENTED_EDGE('',*,*,#9474,.T.);
#13093=ORIENTED_EDGE('',*,*,#9462,.T.);
#13094=ORIENTED_EDGE('',*,*,#9470,.T.);
#13095=ORIENTED_EDGE('',*,*,#9637,.F.);
#13096=ORIENTED_EDGE('',*,*,#9473,.T.);
#13097=ORIENTED_EDGE('',*,*,#9638,.F.);
#13098=ORIENTED_EDGE('',*,*,#9492,.T.);
#13099=ORIENTED_EDGE('',*,*,#9516,.T.);
#13100=ORIENTED_EDGE('',*,*,#9497,.T.);
#13101=ORIENTED_EDGE('',*,*,#9452,.T.);
#13102=ORIENTED_EDGE('',*,*,#9639,.F.);
#13103=ORIENTED_EDGE('',*,*,#9640,.F.);
#13104=ORIENTED_EDGE('',*,*,#9641,.T.);
#13105=ORIENTED_EDGE('',*,*,#9639,.T.);
#13106=ORIENTED_EDGE('',*,*,#9641,.F.);
#13107=ORIENTED_EDGE('',*,*,#9456,.T.);
#13108=ORIENTED_EDGE('',*,*,#9457,.T.);
#13109=ORIENTED_EDGE('',*,*,#9642,.T.);
#13110=ORIENTED_EDGE('',*,*,#9640,.T.);
#13111=ORIENTED_EDGE('',*,*,#9642,.F.);
#13112=ORIENTED_EDGE('',*,*,#9459,.T.);
#13113=ORIENTED_EDGE('',*,*,#9643,.T.);
#13114=ORIENTED_EDGE('',*,*,#9432,.F.);
#13115=ORIENTED_EDGE('',*,*,#9490,.T.);
#13116=ORIENTED_EDGE('',*,*,#9503,.T.);
#13117=ORIENTED_EDGE('',*,*,#9510,.T.);
#13118=ORIENTED_EDGE('',*,*,#9429,.F.);
#13119=ORIENTED_EDGE('',*,*,#9556,.T.);
#13120=ORIENTED_EDGE('',*,*,#9569,.T.);
#13121=ORIENTED_EDGE('',*,*,#9577,.T.);
#13122=ORIENTED_EDGE('',*,*,#9426,.F.);
#13123=ORIENTED_EDGE('',*,*,#9620,.T.);
#13124=ORIENTED_EDGE('',*,*,#9614,.T.);
#13125=ORIENTED_EDGE('',*,*,#9597,.T.);
#13126=ORIENTED_EDGE('',*,*,#9441,.F.);
#13127=ORIENTED_EDGE('',*,*,#9557,.T.);
#13128=ORIENTED_EDGE('',*,*,#9545,.T.);
#13129=ORIENTED_EDGE('',*,*,#9530,.T.);
#13130=ORIENTED_EDGE('',*,*,#9438,.F.);
#13131=ORIENTED_EDGE('',*,*,#9491,.T.);
#13132=ORIENTED_EDGE('',*,*,#9481,.T.);
#13133=ORIENTED_EDGE('',*,*,#9467,.T.);
#13134=ORIENTED_EDGE('',*,*,#9435,.F.);
#13135=ORIENTED_EDGE('',*,*,#9433,.F.);
#13136=ORIENTED_EDGE('',*,*,#9643,.F.);
#13137=ORIENTED_EDGE('',*,*,#9581,.T.);
#13138=ORIENTED_EDGE('',*,*,#9580,.T.);
#13139=ORIENTED_EDGE('',*,*,#9602,.T.);
#13140=ORIENTED_EDGE('',*,*,#9585,.T.);
#13141=ORIENTED_EDGE('',*,*,#9455,.T.);
#13142=ORIENTED_EDGE('',*,*,#9644,.T.);
#13143=ORIENTED_EDGE('',*,*,#9608,.T.);
#13144=ORIENTED_EDGE('',*,*,#9588,.T.);
#13145=ORIENTED_EDGE('',*,*,#9574,.T.);
#13146=ORIENTED_EDGE('',*,*,#9566,.T.);
#13147=ORIENTED_EDGE('',*,*,#9542,.T.);
#13148=ORIENTED_EDGE('',*,*,#9522,.T.);
#13149=ORIENTED_EDGE('',*,*,#9508,.T.);
#13150=ORIENTED_EDGE('',*,*,#9500,.T.);
#13151=ORIENTED_EDGE('',*,*,#9476,.T.);
#13152=ORIENTED_EDGE('',*,*,#9472,.T.);
#13153=ORIENTED_EDGE('',*,*,#9483,.T.);
#13154=ORIENTED_EDGE('',*,*,#9495,.T.);
#13155=ORIENTED_EDGE('',*,*,#9517,.T.);
#13156=ORIENTED_EDGE('',*,*,#9537,.T.);
#13157=ORIENTED_EDGE('',*,*,#9547,.T.);
#13158=ORIENTED_EDGE('',*,*,#9561,.T.);
#13159=ORIENTED_EDGE('',*,*,#9584,.T.);
#13160=ORIENTED_EDGE('',*,*,#9604,.T.);
#13161=ORIENTED_EDGE('',*,*,#9616,.T.);
#13162=ORIENTED_EDGE('',*,*,#9625,.T.);
#13163=ORIENTED_EDGE('',*,*,#9609,.T.);
#13164=ORIENTED_EDGE('',*,*,#9644,.F.);
#13165=ORIENTED_EDGE('',*,*,#9628,.T.);
#13166=ORIENTED_EDGE('',*,*,#9453,.T.);
#13167=ORIENTED_EDGE('',*,*,#9449,.T.);
#13168=ORIENTED_EDGE('',*,*,#9450,.T.);
#13169=ORIENTED_EDGE('',*,*,#9645,.T.);
#13170=ORIENTED_EDGE('',*,*,#9626,.T.);
#13171=ORIENTED_EDGE('',*,*,#9645,.F.);
#13172=ORIENTED_EDGE('',*,*,#9486,.T.);
#13173=ORIENTED_EDGE('',*,*,#9465,.T.);
#13174=ORIENTED_EDGE('',*,*,#9460,.T.);
#13175=ORIENTED_EDGE('',*,*,#9475,.T.);
#13176=ORIENTED_EDGE('',*,*,#9552,.T.);
#13177=ORIENTED_EDGE('',*,*,#9529,.T.);
#13178=ORIENTED_EDGE('',*,*,#9527,.T.);
#13179=ORIENTED_EDGE('',*,*,#9541,.T.);
#13180=ORIENTED_EDGE('',*,*,#9619,.T.);
#13181=ORIENTED_EDGE('',*,*,#9595,.T.);
#13182=ORIENTED_EDGE('',*,*,#9593,.T.);
#13183=ORIENTED_EDGE('',*,*,#9607,.T.);
#13184=ORIENTED_EDGE('',*,*,#9515,.T.);
#13185=ORIENTED_EDGE('',*,*,#9514,.T.);
#13186=ORIENTED_EDGE('',*,*,#9535,.T.);
#13187=ORIENTED_EDGE('',*,*,#9518,.T.);
#16494=PLANE('',#18371);
#16495=PLANE('',#18373);
#16496=PLANE('',#18375);
#16497=PLANE('',#18379);
#16498=PLANE('',#18534);
#16499=PLANE('',#18535);
#16500=PLANE('',#18536);
#16501=PLANE('',#18537);
#16502=PLANE('',#18538);
#16503=PLANE('',#18539);
#16504=PLANE('',#18540);
#16505=PLANE('',#18541);
#16506=PLANE('',#18542);
#16507=PLANE('',#18543);
#16508=PLANE('',#18544);
#16509=PLANE('',#18545);
#16510=PLANE('',#18546);
#16511=PLANE('',#18547);
#16512=PLANE('',#18548);
#16513=PLANE('',#18549);
#16514=PLANE('',#18556);
#16515=PLANE('',#18558);
#16516=PLANE('',#18560);
#16517=PLANE('',#18561);
#16518=PLANE('',#18562);
#16519=PLANE('',#18563);
#17094=ADVANCED_FACE('',(#1759),#387,.T.);
#17095=ADVANCED_FACE('',(#1760),#388,.T.);
#17096=ADVANCED_FACE('',(#1761),#389,.T.);
#17097=ADVANCED_FACE('',(#1762),#390,.T.);
#17098=ADVANCED_FACE('',(#1763),#391,.T.);
#17099=ADVANCED_FACE('',(#1764),#392,.T.);
#17100=ADVANCED_FACE('',(#1765),#393,.T.);
#17101=ADVANCED_FACE('',(#1766),#394,.T.);
#17102=ADVANCED_FACE('',(#1767),#395,.T.);
#17103=ADVANCED_FACE('',(#1768),#396,.T.);
#17104=ADVANCED_FACE('',(#1769),#193,.F.);
#17105=ADVANCED_FACE('',(#1770),#194,.T.);
#17106=ADVANCED_FACE('',(#1771),#195,.F.);
#17107=ADVANCED_FACE('',(#1772),#196,.T.);
#17108=ADVANCED_FACE('',(#1773),#197,.T.);
#17109=ADVANCED_FACE('',(#1774),#198,.T.);
#17110=ADVANCED_FACE('',(#1775),#199,.F.);
#17111=ADVANCED_FACE('',(#1776),#200,.T.);
#17112=ADVANCED_FACE('',(#1777),#201,.T.);
#17113=ADVANCED_FACE('',(#1778),#547,.T.);
#17114=ADVANCED_FACE('',(#1779),#548,.T.);
#17115=ADVANCED_FACE('',(#1780),#168,.T.);
#17116=ADVANCED_FACE('',(#1781,#885),#16494,.F.);
#17117=ADVANCED_FACE('',(#1782),#549,.F.);
#17118=ADVANCED_FACE('',(#1783,#886),#16495,.F.);
#17119=ADVANCED_FACE('',(#1784),#550,.F.);
#17120=ADVANCED_FACE('',(#1785,#887),#16496,.F.);
#17121=ADVANCED_FACE('',(#1786),#551,.T.);
#17122=ADVANCED_FACE('',(#1787),#169,.T.);
#17123=ADVANCED_FACE('',(#1788,#888),#16497,.F.);
#17124=ADVANCED_FACE('',(#1789),#202,.T.);
#17125=ADVANCED_FACE('',(#1790),#203,.F.);
#17126=ADVANCED_FACE('',(#1791),#204,.T.);
#17127=ADVANCED_FACE('',(#1792),#552,.T.);
#17128=ADVANCED_FACE('',(#1793),#397,.T.);
#17129=ADVANCED_FACE('',(#1794),#205,.T.);
#17130=ADVANCED_FACE('',(#1795),#553,.T.);
#17131=ADVANCED_FACE('',(#1796),#554,.T.);
#17132=ADVANCED_FACE('',(#1797),#206,.T.);
#17133=ADVANCED_FACE('',(#1798),#398,.T.);
#17134=ADVANCED_FACE('',(#1799),#207,.T.);
#17135=ADVANCED_FACE('',(#1800),#208,.T.);
#17136=ADVANCED_FACE('',(#1801),#555,.T.);
#17137=ADVANCED_FACE('',(#1802),#556,.T.);
#17138=ADVANCED_FACE('',(#1803),#557,.T.);
#17139=ADVANCED_FACE('',(#1804),#558,.T.);
#17140=ADVANCED_FACE('',(#1805),#559,.T.);
#17141=ADVANCED_FACE('',(#1806),#209,.T.);
#17142=ADVANCED_FACE('',(#1807),#399,.T.);
#17143=ADVANCED_FACE('',(#1808),#210,.T.);
#17144=ADVANCED_FACE('',(#1809),#560,.T.);
#17145=ADVANCED_FACE('',(#1810),#211,.T.);
#17146=ADVANCED_FACE('',(#1811),#561,.T.);
#17147=ADVANCED_FACE('',(#1812),#212,.T.);
#17148=ADVANCED_FACE('',(#1813),#562,.T.);
#17149=ADVANCED_FACE('',(#1814),#400,.T.);
#17150=ADVANCED_FACE('',(#1815),#401,.T.);
#17151=ADVANCED_FACE('',(#1816),#563,.T.);
#17152=ADVANCED_FACE('',(#1817),#213,.T.);
#17153=ADVANCED_FACE('',(#1818),#564,.T.);
#17154=ADVANCED_FACE('',(#1819),#565,.T.);
#17155=ADVANCED_FACE('',(#1820),#566,.T.);
#17156=ADVANCED_FACE('',(#1821),#214,.T.);
#17157=ADVANCED_FACE('',(#1822),#215,.T.);
#17158=ADVANCED_FACE('',(#1823),#216,.T.);
#17159=ADVANCED_FACE('',(#1824),#402,.T.);
#17160=ADVANCED_FACE('',(#1825),#567,.T.);
#17161=ADVANCED_FACE('',(#1826),#568,.T.);
#17162=ADVANCED_FACE('',(#1827),#569,.T.);
#17163=ADVANCED_FACE('',(#1828),#570,.T.);
#17164=ADVANCED_FACE('',(#1829),#571,.T.);
#17165=ADVANCED_FACE('',(#1830),#217,.T.);
#17166=ADVANCED_FACE('',(#1831),#403,.T.);
#17167=ADVANCED_FACE('',(#1832),#218,.T.);
#17168=ADVANCED_FACE('',(#1833),#572,.T.);
#17169=ADVANCED_FACE('',(#1834),#219,.T.);
#17170=ADVANCED_FACE('',(#1835),#573,.T.);
#17171=ADVANCED_FACE('',(#1836),#220,.T.);
#17172=ADVANCED_FACE('',(#1837),#574,.T.);
#17173=ADVANCED_FACE('',(#1838),#404,.T.);
#17174=ADVANCED_FACE('',(#1839),#405,.T.);
#17175=ADVANCED_FACE('',(#1840),#575,.T.);
#17176=ADVANCED_FACE('',(#1841),#221,.T.);
#17177=ADVANCED_FACE('',(#1842),#576,.T.);
#17178=ADVANCED_FACE('',(#1843),#577,.T.);
#17179=ADVANCED_FACE('',(#1844),#578,.T.);
#17180=ADVANCED_FACE('',(#1845),#222,.T.);
#17181=ADVANCED_FACE('',(#1846),#406,.T.);
#17182=ADVANCED_FACE('',(#1847),#223,.T.);
#17183=ADVANCED_FACE('',(#1848),#224,.T.);
#17184=ADVANCED_FACE('',(#1849),#579,.T.);
#17185=ADVANCED_FACE('',(#1850),#580,.T.);
#17186=ADVANCED_FACE('',(#1851),#581,.T.);
#17187=ADVANCED_FACE('',(#1852),#225,.T.);
#17188=ADVANCED_FACE('',(#1853),#16498,.F.);
#17189=ADVANCED_FACE('',(#1854),#16499,.F.);
#17190=ADVANCED_FACE('',(#1855),#16500,.F.);
#17191=ADVANCED_FACE('',(#1856),#16501,.F.);
#17192=ADVANCED_FACE('',(#1857),#16502,.F.);
#17193=ADVANCED_FACE('',(#1858),#16503,.F.);
#17194=ADVANCED_FACE('',(#1859),#16504,.F.);
#17195=ADVANCED_FACE('',(#1860),#16505,.F.);
#17196=ADVANCED_FACE('',(#1861),#16506,.F.);
#17197=ADVANCED_FACE('',(#1862),#16507,.F.);
#17198=ADVANCED_FACE('',(#1863),#16508,.F.);
#17199=ADVANCED_FACE('',(#1864),#16509,.F.);
#17200=ADVANCED_FACE('',(#1865),#16510,.F.);
#17201=ADVANCED_FACE('',(#1866),#16511,.F.);
#17202=ADVANCED_FACE('',(#1867),#16512,.F.);
#17203=ADVANCED_FACE('',(#1868,#889),#16513,.F.);
#17204=ADVANCED_FACE('',(#1869),#226,.T.);
#17205=ADVANCED_FACE('',(#1870),#582,.F.);
#17206=ADVANCED_FACE('',(#1871),#170,.F.);
#17207=ADVANCED_FACE('',(#1872),#16514,.F.);
#17208=ADVANCED_FACE('',(#1873),#583,.T.);
#17209=ADVANCED_FACE('',(#1874,#890),#16515,.F.);
#17210=ADVANCED_FACE('',(#1875),#584,.T.);
#17211=ADVANCED_FACE('',(#1876),#16516,.F.);
#17212=ADVANCED_FACE('',(#1877),#16517,.F.);
#17213=ADVANCED_FACE('',(#1878),#16518,.F.);
#17214=ADVANCED_FACE('',(#1879),#16519,.F.);
#17795=CLOSED_SHELL('',(#17094,#17095,#17096,#17097,#17098,#17099,#17100,
#17101,#17102,#17103,#17104,#17105,#17106,#17107,#17108,#17109,#17110,#17111,
#17112,#17113,#17114,#17115,#17116,#17117,#17118,#17119,#17120,#17121,#17122,
#17123,#17124,#17125,#17126,#17127,#17128,#17129,#17130,#17131,#17132,#17133,
#17134,#17135,#17136,#17137,#17138,#17139,#17140,#17141,#17142,#17143,#17144,
#17145,#17146,#17147,#17148,#17149,#17150,#17151,#17152,#17153,#17154,#17155,
#17156,#17157,#17158,#17159,#17160,#17161,#17162,#17163,#17164,#17165,#17166,
#17167,#17168,#17169,#17170,#17171,#17172,#17173,#17174,#17175,#17176,#17177,
#17178,#17179,#17180,#17181,#17182,#17183,#17184,#17185,#17186,#17187,#17188,
#17189,#17190,#17191,#17192,#17193,#17194,#17195,#17196,#17197,#17198,#17199,
#17200,#17201,#17202,#17203,#17204,#17205,#17206,#17207,#17208,#17209,#17210,
#17211,#17212,#17213,#17214));
#18270=AXIS2_PLACEMENT_3D('',#25558,#20700,#20701);
#18271=AXIS2_PLACEMENT_3D('',#25559,#20702,#20703);
#18272=AXIS2_PLACEMENT_3D('',#25562,#20704,#20705);
#18273=AXIS2_PLACEMENT_3D('',#25564,#20706,#20707);
#18274=AXIS2_PLACEMENT_3D('',#25565,#20708,#20709);
#18275=AXIS2_PLACEMENT_3D('',#25566,#20710,#20711);
#18276=AXIS2_PLACEMENT_3D('',#25569,#20712,#20713);
#18277=AXIS2_PLACEMENT_3D('',#25571,#20714,#20715);
#18278=AXIS2_PLACEMENT_3D('',#25572,#20716,#20717);
#18279=AXIS2_PLACEMENT_3D('',#25573,#20718,#20719);
#18280=AXIS2_PLACEMENT_3D('',#25576,#20720,#20721);
#18281=AXIS2_PLACEMENT_3D('',#25578,#20722,#20723);
#18282=AXIS2_PLACEMENT_3D('',#25580,#20724,#20725);
#18283=AXIS2_PLACEMENT_3D('',#25593,#20726,#20727);
#18284=AXIS2_PLACEMENT_3D('',#25596,#20728,#20729);
#18285=AXIS2_PLACEMENT_3D('',#25598,#20730,#20731);
#18286=AXIS2_PLACEMENT_3D('',#25599,#20732,#20733);
#18287=AXIS2_PLACEMENT_3D('',#25600,#20734,#20735);
#18288=AXIS2_PLACEMENT_3D('',#25603,#20736,#20737);
#18289=AXIS2_PLACEMENT_3D('',#25605,#20738,#20739);
#18290=AXIS2_PLACEMENT_3D('',#25607,#20740,#20741);
#18291=AXIS2_PLACEMENT_3D('',#25620,#20742,#20743);
#18292=AXIS2_PLACEMENT_3D('',#25623,#20744,#20745);
#18293=AXIS2_PLACEMENT_3D('',#25625,#20746,#20747);
#18294=AXIS2_PLACEMENT_3D('',#25626,#20748,#20749);
#18295=AXIS2_PLACEMENT_3D('',#25627,#20750,#20751);
#18296=AXIS2_PLACEMENT_3D('',#25630,#20752,#20753);
#18297=AXIS2_PLACEMENT_3D('',#25632,#20754,#20755);
#18298=AXIS2_PLACEMENT_3D('',#25646,#20756,#20757);
#18299=AXIS2_PLACEMENT_3D('',#25647,#20758,#20759);
#18300=AXIS2_PLACEMENT_3D('',#25650,#20760,#20761);
#18301=AXIS2_PLACEMENT_3D('',#25665,#20762,#20763);
#18302=AXIS2_PLACEMENT_3D('',#25666,#20764,#20765);
#18303=AXIS2_PLACEMENT_3D('',#25667,#20766,#20767);
#18304=AXIS2_PLACEMENT_3D('',#25670,#20768,#20769);
#18305=AXIS2_PLACEMENT_3D('',#25672,#20770,#20771);
#18306=AXIS2_PLACEMENT_3D('',#25673,#20772,#20773);
#18307=AXIS2_PLACEMENT_3D('',#25674,#20774,#20775);
#18308=AXIS2_PLACEMENT_3D('',#25677,#20776,#20777);
#18309=AXIS2_PLACEMENT_3D('',#25679,#20778,#20779);
#18310=AXIS2_PLACEMENT_3D('',#25680,#20780,#20781);
#18311=AXIS2_PLACEMENT_3D('',#25681,#20782,#20783);
#18312=AXIS2_PLACEMENT_3D('',#25683,#20784,#20785);
#18313=AXIS2_PLACEMENT_3D('',#25685,#20786,#20787);
#18314=AXIS2_PLACEMENT_3D('',#25686,#20788,#20789);
#18315=AXIS2_PLACEMENT_3D('',#25687,#20790,#20791);
#18316=AXIS2_PLACEMENT_3D('',#25690,#20792,#20793);
#18317=AXIS2_PLACEMENT_3D('',#25691,#20794,#20795);
#18318=AXIS2_PLACEMENT_3D('',#25693,#20796,#20797);
#18319=AXIS2_PLACEMENT_3D('',#25694,#20798,#20799);
#18320=AXIS2_PLACEMENT_3D('',#25695,#20800,#20801);
#18321=AXIS2_PLACEMENT_3D('',#25697,#20802,#20803);
#18322=AXIS2_PLACEMENT_3D('',#25699,#20804,#20805);
#18323=AXIS2_PLACEMENT_3D('',#25701,#20806,#20807);
#18324=AXIS2_PLACEMENT_3D('',#25702,#20808,#20809);
#18325=AXIS2_PLACEMENT_3D('',#25703,#20810,#20811);
#18326=AXIS2_PLACEMENT_3D('',#25705,#20812,#20813);
#18327=AXIS2_PLACEMENT_3D('',#25707,#20814,#20815);
#18328=AXIS2_PLACEMENT_3D('',#25708,#20816,#20817);
#18329=AXIS2_PLACEMENT_3D('',#25709,#20818,#20819);
#18330=AXIS2_PLACEMENT_3D('',#25711,#20820,#20821);
#18331=AXIS2_PLACEMENT_3D('',#25713,#20822,#20823);
#18332=AXIS2_PLACEMENT_3D('',#25715,#20824,#20825);
#18333=AXIS2_PLACEMENT_3D('',#25716,#20826,#20827);
#18334=AXIS2_PLACEMENT_3D('',#25717,#20828,#20829);
#18335=AXIS2_PLACEMENT_3D('',#25719,#20830,#20831);
#18336=AXIS2_PLACEMENT_3D('',#25721,#20832,#20833);
#18337=AXIS2_PLACEMENT_3D('',#25722,#20834,#20835);
#18338=AXIS2_PLACEMENT_3D('',#25723,#20836,#20837);
#18339=AXIS2_PLACEMENT_3D('',#25725,#20838,#20839);
#18340=AXIS2_PLACEMENT_3D('',#25727,#20840,#20841);
#18341=AXIS2_PLACEMENT_3D('',#25728,#20842,#20843);
#18342=AXIS2_PLACEMENT_3D('',#25729,#20844,#20845);
#18343=AXIS2_PLACEMENT_3D('',#25731,#20846,#20847);
#18344=AXIS2_PLACEMENT_3D('',#25733,#20848,#20849);
#18345=AXIS2_PLACEMENT_3D('',#25734,#20850,#20851);
#18346=AXIS2_PLACEMENT_3D('',#25735,#20852,#20853);
#18347=AXIS2_PLACEMENT_3D('',#25737,#20854,#20855);
#18348=AXIS2_PLACEMENT_3D('',#25739,#20856,#20857);
#18349=AXIS2_PLACEMENT_3D('',#25740,#20858,#20859);
#18350=AXIS2_PLACEMENT_3D('',#25741,#20860,#20861);
#18351=AXIS2_PLACEMENT_3D('',#25743,#20863,#20864);
#18352=AXIS2_PLACEMENT_3D('',#25747,#20866,#20867);
#18353=AXIS2_PLACEMENT_3D('',#25769,#20868,#20869);
#18354=AXIS2_PLACEMENT_3D('',#25776,#20870,#20871);
#18355=AXIS2_PLACEMENT_3D('',#25785,#20872,#20873);
#18356=AXIS2_PLACEMENT_3D('',#25807,#20874,#20875);
#18357=AXIS2_PLACEMENT_3D('',#25829,#20876,#20877);
#18358=AXIS2_PLACEMENT_3D('',#25837,#20878,#20879);
#18359=AXIS2_PLACEMENT_3D('',#25859,#20880,#20881);
#18360=AXIS2_PLACEMENT_3D('',#25880,#20882,#20883);
#18361=AXIS2_PLACEMENT_3D('',#25889,#20884,#20885);
#18362=AXIS2_PLACEMENT_3D('',#25910,#20886,#20887);
#18363=AXIS2_PLACEMENT_3D('',#25911,#20888,#20889);
#18364=AXIS2_PLACEMENT_3D('',#25914,#20890,#20891);
#18365=AXIS2_PLACEMENT_3D('',#25961,#20892,#20893);
#18366=AXIS2_PLACEMENT_3D('',#26008,#20894,#20895);
#18367=AXIS2_PLACEMENT_3D('',#26010,#20896,#20897);
#18368=AXIS2_PLACEMENT_3D('',#26013,#20899,#20900);
#18369=AXIS2_PLACEMENT_3D('',#26060,#20901,#20902);
#18370=AXIS2_PLACEMENT_3D('',#26107,#20903,#20904);
#18371=AXIS2_PLACEMENT_3D('',#26152,#20905,#20906);
#18372=AXIS2_PLACEMENT_3D('',#26153,#20907,#20908);
#18373=AXIS2_PLACEMENT_3D('',#26155,#20910,#20911);
#18374=AXIS2_PLACEMENT_3D('',#26156,#20912,#20913);
#18375=AXIS2_PLACEMENT_3D('',#26158,#20915,#20916);
#18376=AXIS2_PLACEMENT_3D('',#26160,#20917,#20918);
#18377=AXIS2_PLACEMENT_3D('',#26161,#20919,#20920);
#18378=AXIS2_PLACEMENT_3D('',#26163,#20922,#20923);
#18379=AXIS2_PLACEMENT_3D('',#26165,#20925,#20926);
#18380=AXIS2_PLACEMENT_3D('',#26166,#20927,#20928);
#18381=AXIS2_PLACEMENT_3D('',#26169,#20929,#20930);
#18382=AXIS2_PLACEMENT_3D('',#26170,#20931,#20932);
#18383=AXIS2_PLACEMENT_3D('',#26172,#20933,#20934);
#18384=AXIS2_PLACEMENT_3D('',#26173,#20935,#20936);
#18385=AXIS2_PLACEMENT_3D('',#26174,#20937,#20938);
#18386=AXIS2_PLACEMENT_3D('',#26176,#20939,#20940);
#18387=AXIS2_PLACEMENT_3D('',#26178,#20941,#20942);
#18388=AXIS2_PLACEMENT_3D('',#26179,#20943,#20944);
#18389=AXIS2_PLACEMENT_3D('',#26180,#20945,#20946);
#18390=AXIS2_PLACEMENT_3D('',#26183,#20947,#20948);
#18391=AXIS2_PLACEMENT_3D('',#26184,#20949,#20950);
#18392=AXIS2_PLACEMENT_3D('',#26186,#20951,#20952);
#18393=AXIS2_PLACEMENT_3D('',#26187,#20953,#20954);
#18394=AXIS2_PLACEMENT_3D('',#26188,#20955,#20956);
#18395=AXIS2_PLACEMENT_3D('',#26192,#20958,#20959);
#18396=AXIS2_PLACEMENT_3D('',#26194,#20961,#20962);
#18397=AXIS2_PLACEMENT_3D('',#26195,#20963,#20964);
#18398=AXIS2_PLACEMENT_3D('',#26196,#20965,#20966);
#18399=AXIS2_PLACEMENT_3D('',#26197,#20967,#20968);
#18400=AXIS2_PLACEMENT_3D('',#26199,#20969,#20970);
#18401=AXIS2_PLACEMENT_3D('',#26200,#20971,#20972);
#18402=AXIS2_PLACEMENT_3D('',#26201,#20973,#20974);
#18403=AXIS2_PLACEMENT_3D('',#26222,#20978,#20979);
#18404=AXIS2_PLACEMENT_3D('',#26244,#20982,#20983);
#18405=AXIS2_PLACEMENT_3D('',#26245,#20984,#20985);
#18406=AXIS2_PLACEMENT_3D('',#26246,#20986,#20987);
#18407=AXIS2_PLACEMENT_3D('',#26247,#20988,#20989);
#18408=AXIS2_PLACEMENT_3D('',#26248,#20990,#20991);
#18409=AXIS2_PLACEMENT_3D('',#26250,#20992,#20993);
#18410=AXIS2_PLACEMENT_3D('',#26251,#20994,#20995);
#18411=AXIS2_PLACEMENT_3D('',#26252,#20996,#20997);
#18412=AXIS2_PLACEMENT_3D('',#26271,#20998,#20999);
#18413=AXIS2_PLACEMENT_3D('',#26272,#21000,#21001);
#18414=AXIS2_PLACEMENT_3D('',#26273,#21002,#21003);
#18415=AXIS2_PLACEMENT_3D('',#26292,#21004,#21005);
#18416=AXIS2_PLACEMENT_3D('',#26293,#21006,#21007);
#18417=AXIS2_PLACEMENT_3D('',#26294,#21008,#21009);
#18418=AXIS2_PLACEMENT_3D('',#26297,#21012,#21013);
#18419=AXIS2_PLACEMENT_3D('',#26320,#21017,#21018);
#18420=AXIS2_PLACEMENT_3D('',#26325,#21022,#21023);
#18421=AXIS2_PLACEMENT_3D('',#26328,#21024,#21025);
#18422=AXIS2_PLACEMENT_3D('',#26331,#21027,#21028);
#18423=AXIS2_PLACEMENT_3D('',#26333,#21030,#21031);
#18424=AXIS2_PLACEMENT_3D('',#26336,#21032,#21033);
#18425=AXIS2_PLACEMENT_3D('',#26356,#21036,#21037);
#18426=AXIS2_PLACEMENT_3D('',#26373,#21038,#21039);
#18427=AXIS2_PLACEMENT_3D('',#26374,#21040,#21041);
#18428=AXIS2_PLACEMENT_3D('',#26375,#21042,#21043);
#18429=AXIS2_PLACEMENT_3D('',#26377,#21044,#21045);
#18430=AXIS2_PLACEMENT_3D('',#26378,#21046,#21047);
#18431=AXIS2_PLACEMENT_3D('',#26379,#21048,#21049);
#18432=AXIS2_PLACEMENT_3D('',#26381,#21050,#21051);
#18433=AXIS2_PLACEMENT_3D('',#26383,#21052,#21053);
#18434=AXIS2_PLACEMENT_3D('',#26400,#21054,#21055);
#18435=AXIS2_PLACEMENT_3D('',#26405,#21059,#21060);
#18436=AXIS2_PLACEMENT_3D('',#26407,#21061,#21062);
#18437=AXIS2_PLACEMENT_3D('',#26408,#21063,#21064);
#18438=AXIS2_PLACEMENT_3D('',#26409,#21065,#21066);
#18439=AXIS2_PLACEMENT_3D('',#26412,#21069,#21070);
#18440=AXIS2_PLACEMENT_3D('',#26413,#21071,#21072);
#18441=AXIS2_PLACEMENT_3D('',#26414,#21073,#21074);
#18442=AXIS2_PLACEMENT_3D('',#26415,#21075,#21076);
#18443=AXIS2_PLACEMENT_3D('',#26418,#21077,#21078);
#18444=AXIS2_PLACEMENT_3D('',#26421,#21080,#21081);
#18445=AXIS2_PLACEMENT_3D('',#26423,#21083,#21084);
#18446=AXIS2_PLACEMENT_3D('',#26425,#21085,#21086);
#18447=AXIS2_PLACEMENT_3D('',#26426,#21087,#21088);
#18448=AXIS2_PLACEMENT_3D('',#26427,#21089,#21090);
#18449=AXIS2_PLACEMENT_3D('',#26429,#21091,#21092);
#18450=AXIS2_PLACEMENT_3D('',#26430,#21093,#21094);
#18451=AXIS2_PLACEMENT_3D('',#26431,#21095,#21096);
#18452=AXIS2_PLACEMENT_3D('',#26434,#21099,#21100);
#18453=AXIS2_PLACEMENT_3D('',#26435,#21101,#21102);
#18454=AXIS2_PLACEMENT_3D('',#26436,#21103,#21104);
#18455=AXIS2_PLACEMENT_3D('',#26457,#21108,#21109);
#18456=AXIS2_PLACEMENT_3D('',#26460,#21112,#21113);
#18457=AXIS2_PLACEMENT_3D('',#26482,#21116,#21117);
#18458=AXIS2_PLACEMENT_3D('',#26483,#21118,#21119);
#18459=AXIS2_PLACEMENT_3D('',#26486,#21120,#21121);
#18460=AXIS2_PLACEMENT_3D('',#26487,#21122,#21123);
#18461=AXIS2_PLACEMENT_3D('',#26488,#21124,#21125);
#18462=AXIS2_PLACEMENT_3D('',#26489,#21126,#21127);
#18463=AXIS2_PLACEMENT_3D('',#26508,#21128,#21129);
#18464=AXIS2_PLACEMENT_3D('',#26509,#21130,#21131);
#18465=AXIS2_PLACEMENT_3D('',#26510,#21132,#21133);
#18466=AXIS2_PLACEMENT_3D('',#26529,#21134,#21135);
#18467=AXIS2_PLACEMENT_3D('',#26530,#21136,#21137);
#18468=AXIS2_PLACEMENT_3D('',#26531,#21138,#21139);
#18469=AXIS2_PLACEMENT_3D('',#26533,#21140,#21141);
#18470=AXIS2_PLACEMENT_3D('',#26534,#21142,#21143);
#18471=AXIS2_PLACEMENT_3D('',#26535,#21144,#21145);
#18472=AXIS2_PLACEMENT_3D('',#26538,#21148,#21149);
#18473=AXIS2_PLACEMENT_3D('',#26561,#21153,#21154);
#18474=AXIS2_PLACEMENT_3D('',#26564,#21156,#21157);
#18475=AXIS2_PLACEMENT_3D('',#26568,#21160,#21161);
#18476=AXIS2_PLACEMENT_3D('',#26571,#21163,#21164);
#18477=AXIS2_PLACEMENT_3D('',#26573,#21166,#21167);
#18478=AXIS2_PLACEMENT_3D('',#26576,#21168,#21169);
#18479=AXIS2_PLACEMENT_3D('',#26596,#21172,#21173);
#18480=AXIS2_PLACEMENT_3D('',#26613,#21174,#21175);
#18481=AXIS2_PLACEMENT_3D('',#26614,#21176,#21177);
#18482=AXIS2_PLACEMENT_3D('',#26615,#21178,#21179);
#18483=AXIS2_PLACEMENT_3D('',#26617,#21180,#21181);
#18484=AXIS2_PLACEMENT_3D('',#26618,#21182,#21183);
#18485=AXIS2_PLACEMENT_3D('',#26619,#21184,#21185);
#18486=AXIS2_PLACEMENT_3D('',#26621,#21186,#21187);
#18487=AXIS2_PLACEMENT_3D('',#26623,#21188,#21189);
#18488=AXIS2_PLACEMENT_3D('',#26640,#21190,#21191);
#18489=AXIS2_PLACEMENT_3D('',#26642,#21192,#21193);
#18490=AXIS2_PLACEMENT_3D('',#26647,#21197,#21198);
#18491=AXIS2_PLACEMENT_3D('',#26648,#21199,#21200);
#18492=AXIS2_PLACEMENT_3D('',#26649,#21201,#21202);
#18493=AXIS2_PLACEMENT_3D('',#26652,#21205,#21206);
#18494=AXIS2_PLACEMENT_3D('',#26655,#21207,#21208);
#18495=AXIS2_PLACEMENT_3D('',#26656,#21209,#21210);
#18496=AXIS2_PLACEMENT_3D('',#26657,#21211,#21212);
#18497=AXIS2_PLACEMENT_3D('',#26658,#21213,#21214);
#18498=AXIS2_PLACEMENT_3D('',#26661,#21216,#21217);
#18499=AXIS2_PLACEMENT_3D('',#26663,#21219,#21220);
#18500=AXIS2_PLACEMENT_3D('',#26665,#21221,#21222);
#18501=AXIS2_PLACEMENT_3D('',#26666,#21223,#21224);
#18502=AXIS2_PLACEMENT_3D('',#26667,#21225,#21226);
#18503=AXIS2_PLACEMENT_3D('',#26669,#21227,#21228);
#18504=AXIS2_PLACEMENT_3D('',#26670,#21229,#21230);
#18505=AXIS2_PLACEMENT_3D('',#26671,#21231,#21232);
#18506=AXIS2_PLACEMENT_3D('',#26674,#21235,#21236);
#18507=AXIS2_PLACEMENT_3D('',#26676,#21237,#21238);
#18508=AXIS2_PLACEMENT_3D('',#26677,#21239,#21240);
#18509=AXIS2_PLACEMENT_3D('',#26678,#21241,#21242);
#18510=AXIS2_PLACEMENT_3D('',#26699,#21246,#21247);
#18511=AXIS2_PLACEMENT_3D('',#26702,#21250,#21251);
#18512=AXIS2_PLACEMENT_3D('',#26724,#21254,#21255);
#18513=AXIS2_PLACEMENT_3D('',#26725,#21256,#21257);
#18514=AXIS2_PLACEMENT_3D('',#26726,#21258,#21259);
#18515=AXIS2_PLACEMENT_3D('',#26728,#21260,#21261);
#18516=AXIS2_PLACEMENT_3D('',#26729,#21262,#21263);
#18517=AXIS2_PLACEMENT_3D('',#26730,#21264,#21265);
#18518=AXIS2_PLACEMENT_3D('',#26732,#21266,#21267);
#18519=AXIS2_PLACEMENT_3D('',#26733,#21268,#21269);
#18520=AXIS2_PLACEMENT_3D('',#26734,#21270,#21271);
#18521=AXIS2_PLACEMENT_3D('',#26753,#21272,#21273);
#18522=AXIS2_PLACEMENT_3D('',#26754,#21274,#21275);
#18523=AXIS2_PLACEMENT_3D('',#26755,#21276,#21277);
#18524=AXIS2_PLACEMENT_3D('',#26774,#21278,#21279);
#18525=AXIS2_PLACEMENT_3D('',#26775,#21280,#21281);
#18526=AXIS2_PLACEMENT_3D('',#26776,#21282,#21283);
#18527=AXIS2_PLACEMENT_3D('',#26779,#21286,#21287);
#18528=AXIS2_PLACEMENT_3D('',#26784,#21291,#21292);
#18529=AXIS2_PLACEMENT_3D('',#26786,#21293,#21294);
#18530=AXIS2_PLACEMENT_3D('',#26789,#21297,#21298);
#18531=AXIS2_PLACEMENT_3D('',#26791,#21299,#21300);
#18532=AXIS2_PLACEMENT_3D('',#26793,#21301,#21302);
#18533=AXIS2_PLACEMENT_3D('',#26794,#21303,#21304);
#18534=AXIS2_PLACEMENT_3D('',#26795,#21305,#21306);
#18535=AXIS2_PLACEMENT_3D('',#26798,#21309,#21310);
#18536=AXIS2_PLACEMENT_3D('',#26799,#21311,#21312);
#18537=AXIS2_PLACEMENT_3D('',#26800,#21313,#21314);
#18538=AXIS2_PLACEMENT_3D('',#26803,#21317,#21318);
#18539=AXIS2_PLACEMENT_3D('',#26804,#21319,#21320);
#18540=AXIS2_PLACEMENT_3D('',#26805,#21321,#21322);
#18541=AXIS2_PLACEMENT_3D('',#26808,#21325,#21326);
#18542=AXIS2_PLACEMENT_3D('',#26809,#21327,#21328);
#18543=AXIS2_PLACEMENT_3D('',#26810,#21329,#21330);
#18544=AXIS2_PLACEMENT_3D('',#26813,#21333,#21334);
#18545=AXIS2_PLACEMENT_3D('',#26814,#21335,#21336);
#18546=AXIS2_PLACEMENT_3D('',#26815,#21337,#21338);
#18547=AXIS2_PLACEMENT_3D('',#26818,#21341,#21342);
#18548=AXIS2_PLACEMENT_3D('',#26819,#21343,#21344);
#18549=AXIS2_PLACEMENT_3D('',#26820,#21345,#21346);
#18550=AXIS2_PLACEMENT_3D('',#26822,#21347,#21348);
#18551=AXIS2_PLACEMENT_3D('',#26823,#21349,#21350);
#18552=AXIS2_PLACEMENT_3D('',#26825,#21351,#21352);
#18553=AXIS2_PLACEMENT_3D('',#26826,#21353,#21354);
#18554=AXIS2_PLACEMENT_3D('',#26827,#21355,#21356);
#18555=AXIS2_PLACEMENT_3D('',#26829,#21358,#21359);
#18556=AXIS2_PLACEMENT_3D('',#26831,#21361,#21362);
#18557=AXIS2_PLACEMENT_3D('',#26832,#21363,#21364);
#18558=AXIS2_PLACEMENT_3D('',#26834,#21366,#21367);
#18559=AXIS2_PLACEMENT_3D('',#26835,#21368,#21369);
#18560=AXIS2_PLACEMENT_3D('',#26837,#21371,#21372);
#18561=AXIS2_PLACEMENT_3D('',#26838,#21373,#21374);
#18562=AXIS2_PLACEMENT_3D('',#26839,#21375,#21376);
#18563=AXIS2_PLACEMENT_3D('',#26840,#21377,#21378);
#20700=DIRECTION('axis',(0.,0.,1.));
#20701=DIRECTION('refdir',(1.,0.,0.));
#20702=DIRECTION('center_axis',(-0.236333478439914,-0.971672005858196,0.));
#20703=DIRECTION('ref_axis',(0.,0.,1.));
#20704=DIRECTION('center_axis',(0.0754966680796046,-0.997146054050698,-2.74692391220027E-14));
#20705=DIRECTION('ref_axis',(0.997146054050698,0.0754966680796046,1.5942911265521E-28));
#20706=DIRECTION('center_axis',(-0.999339812484074,-0.0363309672909394,
0.));
#20707=DIRECTION('ref_axis',(-0.0363309672909394,0.999339812484074,0.));
#20708=DIRECTION('center_axis',(0.,0.,1.));
#20709=DIRECTION('ref_axis',(-0.236333478439928,-0.971672005858193,0.));
#20710=DIRECTION('center_axis',(-0.23633347843992,-0.971672005858195,0.));
#20711=DIRECTION('ref_axis',(0.,0.,1.));
#20712=DIRECTION('center_axis',(0.,0.,-1.));
#20713=DIRECTION('ref_axis',(-0.236333478439908,-0.971672005858198,0.));
#20714=DIRECTION('center_axis',(-0.415306904260248,0.909681359198796,-5.45231211346703E-15));
#20715=DIRECTION('ref_axis',(-0.909681359198796,-0.415306904260248,1.26922783649562E-28));
#20716=DIRECTION('center_axis',(-0.925012498947632,-0.379936674711269,0.));
#20717=DIRECTION('ref_axis',(0.37993667471127,-0.925012498947632,0.));
#20718=DIRECTION('center_axis',(-0.236333478439914,-0.971672005858196,0.));
#20719=DIRECTION('ref_axis',(0.,0.,1.));
#20720=DIRECTION('center_axis',(0.0028764021739081,-0.0379909888811286,
0.999273941957043));
#20721=DIRECTION('ref_axis',(-0.236178256038945,-0.971033817554429,-0.0362375018464822));
#20722=DIRECTION('center_axis',(-0.0754966680796046,0.997146054050698,-2.85413571912387E-14));
#20723=DIRECTION('ref_axis',(-0.997146054050698,-0.0754966680796046,1.65546549913322E-28));
#20724=DIRECTION('center_axis',(0.993204169284826,0.11638504248931,0.));
#20725=DIRECTION('ref_axis',(0.11638504248931,-0.993204169284826,0.));
#20726=DIRECTION('center_axis',(-0.23633347843992,-0.971672005858195,0.));
#20727=DIRECTION('ref_axis',(0.,0.,1.));
#20728=DIRECTION('center_axis',(0.971672005858197,-0.236333478439911,0.));
#20729=DIRECTION('ref_axis',(0.236333478439911,0.971672005858197,0.));
#20730=DIRECTION('center_axis',(0.274011388509925,0.961726447055951,0.));
#20731=DIRECTION('ref_axis',(-0.961726447055951,0.274011388509925,0.));
#20732=DIRECTION('center_axis',(0.,0.,-1.));
#20733=DIRECTION('ref_axis',(-0.236333478439934,-0.971672005858191,0.));
#20734=DIRECTION('center_axis',(-0.23633347843992,-0.971672005858195,0.));
#20735=DIRECTION('ref_axis',(0.,0.,1.));
#20736=DIRECTION('center_axis',(-0.34095089927767,0.940081105161543,-9.65676829998355E-15));
#20737=DIRECTION('ref_axis',(0.940081105161543,0.34095089927767,-1.40353996739024E-28));
#20738=DIRECTION('center_axis',(0.92501249894764,0.379936674711252,0.));
#20739=DIRECTION('ref_axis',(-0.379936674711251,0.925012498947639,0.));
#20740=DIRECTION('center_axis',(-0.0352437692312558,-0.0144759130295536,
0.999273898724636));
#20741=DIRECTION('ref_axis',(0.971210055190269,-0.236221121175772,0.0308319737898077));
#20742=DIRECTION('center_axis',(-0.23633347843992,-0.971672005858195,0.));
#20743=DIRECTION('ref_axis',(0.,0.,1.));
#20744=DIRECTION('center_axis',(0.198296686754741,0.980142042778542,-9.74044619800714E-16));
#20745=DIRECTION('ref_axis',(0.980142042778542,-0.198296686754741,-1.3764509829553E-29));
#20746=DIRECTION('center_axis',(0.971672005858197,-0.236333478439911,0.));
#20747=DIRECTION('ref_axis',(0.236333478439911,0.971672005858197,0.));
#20748=DIRECTION('center_axis',(0.,0.,1.));
#20749=DIRECTION('ref_axis',(-0.236333478439934,-0.971672005858191,0.));
#20750=DIRECTION('center_axis',(-0.23633347843992,-0.971672005858195,0.));
#20751=DIRECTION('ref_axis',(0.,0.,1.));
#20752=DIRECTION('center_axis',(0.647185832447714,-0.762332275506527,-2.49982082791546E-14));
#20753=DIRECTION('ref_axis',(0.762332275506527,0.647185832447714,1.52661900852052E-28));
#20754=DIRECTION('center_axis',(0.735109640272731,0.677948240486024,0.));
#20755=DIRECTION('ref_axis',(-0.677948240486024,0.735109640272731,0.));
#20756=DIRECTION('center_axis',(0.0246576012256848,-0.0290446488604601,
-0.999273941957043));
#20757=DIRECTION('ref_axis',(0.971210082705378,-0.236221127868081,0.0308310557740814));
#20758=DIRECTION('center_axis',(-0.23633347843992,-0.971672005858195,0.));
#20759=DIRECTION('ref_axis',(0.,0.,1.));
#20760=DIRECTION('center_axis',(-0.0200037109101314,-0.0324264290370445,
-0.999273925532799));
#20761=DIRECTION('ref_axis',(-0.23617825252725,-0.971033803116402,0.0362379116185114));
#20762=DIRECTION('center_axis',(-0.828649631183008,0.559767620303519,3.15597567973487E-15));
#20763=DIRECTION('ref_axis',(-0.559767620303519,-0.828649631183008,-6.36709701349244E-32));
#20764=DIRECTION('center_axis',(-0.525029657457571,-0.851083931695333,0.));
#20765=DIRECTION('ref_axis',(0.851083931695333,-0.525029657457571,0.));
#20766=DIRECTION('center_axis',(-0.23633347843992,-0.971672005858195,0.));
#20767=DIRECTION('ref_axis',(0.,0.,1.));
#20768=DIRECTION('center_axis',(0.,0.,1.));
#20769=DIRECTION('ref_axis',(-0.236333478439934,-0.971672005858191,0.));
#20770=DIRECTION('center_axis',(-0.647185832447714,0.762332275506527,0.));
#20771=DIRECTION('ref_axis',(-0.762332275506527,-0.647185832447714,0.));
#20772=DIRECTION('center_axis',(0.787128084679879,0.616789573767412,0.));
#20773=DIRECTION('ref_axis',(0.616789573767412,-0.787128084679879,0.));
#20774=DIRECTION('center_axis',(-0.23633347843992,-0.971672005858195,0.));
#20775=DIRECTION('ref_axis',(0.,0.,1.));
#20776=DIRECTION('center_axis',(0.870893430543957,-0.491471904217706,3.3389056492716E-15));
#20777=DIRECTION('ref_axis',(0.491471904217706,0.870893430543957,-1.97739864827934E-29));
#20778=DIRECTION('center_axis',(-0.525029657457559,-0.85108393169534,0.));
#20779=DIRECTION('ref_axis',(-0.85108393169534,0.525029657457559,0.));
#20780=DIRECTION('center_axis',(0.,0.,1.));
#20781=DIRECTION('ref_axis',(-0.236333478439934,-0.971672005858191,0.));
#20782=DIRECTION('center_axis',(0.,0.,1.));
#20783=DIRECTION('ref_axis',(-0.330288866442325,-0.943879899512774,0.));
#20784=DIRECTION('center_axis',(0.,0.,1.));
#20785=DIRECTION('ref_axis',(-0.330288866442324,-0.943879899512774,0.));
#20786=DIRECTION('center_axis',(0.943879899512774,-0.330288866442324,0.));
#20787=DIRECTION('ref_axis',(0.330288866442324,0.943879899512774,0.));
#20788=DIRECTION('center_axis',(0.,0.,-1.));
#20789=DIRECTION('ref_axis',(-0.330288866442325,-0.943879899512774,0.));
#20790=DIRECTION('center_axis',(0.,0.,-1.));
#20791=DIRECTION('ref_axis',(0.330288866442325,0.943879899512774,0.));
#20792=DIRECTION('center_axis',(0.,0.,-1.));
#20793=DIRECTION('ref_axis',(0.330288866442324,0.943879899512774,0.));
#20794=DIRECTION('center_axis',(0.,0.,-1.));
#20795=DIRECTION('ref_axis',(0.330288866442324,0.943879899512774,0.));
#20796=DIRECTION('center_axis',(-0.943879899512774,0.330288866442325,0.));
#20797=DIRECTION('ref_axis',(-0.330288866442325,-0.943879899512774,0.));
#20798=DIRECTION('center_axis',(0.,0.,1.));
#20799=DIRECTION('ref_axis',(-0.330288866442324,-0.943879899512774,0.));
#20800=DIRECTION('center_axis',(0.,0.,1.));
#20801=DIRECTION('ref_axis',(-0.330288866442324,-0.943879899512774,0.));
#20802=DIRECTION('center_axis',(0.,0.,1.));
#20803=DIRECTION('ref_axis',(-0.330288866442324,-0.943879899512774,0.));
#20804=DIRECTION('center_axis',(0.943879899512774,-0.330288866442324,0.));
#20805=DIRECTION('ref_axis',(0.330288866442324,0.943879899512774,0.));
#20806=DIRECTION('center_axis',(0.,0.,-1.));
#20807=DIRECTION('ref_axis',(0.330288866442325,0.943879899512774,0.));
#20808=DIRECTION('center_axis',(0.,0.,-1.));
#20809=DIRECTION('ref_axis',(0.330288866442325,0.943879899512774,0.));
#20810=DIRECTION('center_axis',(0.,0.,1.));
#20811=DIRECTION('ref_axis',(-0.330288866442324,-0.943879899512774,0.));
#20812=DIRECTION('center_axis',(0.,0.,1.));
#20813=DIRECTION('ref_axis',(-0.330288866442324,-0.943879899512774,0.));
#20814=DIRECTION('center_axis',(-0.943879899512774,0.330288866442325,0.));
#20815=DIRECTION('ref_axis',(0.330288866442325,0.943879899512774,0.));
#20816=DIRECTION('center_axis',(0.,0.,-1.));
#20817=DIRECTION('ref_axis',(-0.330288866442325,-0.943879899512774,0.));
#20818=DIRECTION('center_axis',(0.,0.,-1.));
#20819=DIRECTION('ref_axis',(0.330288866442324,0.943879899512774,0.));
#20820=DIRECTION('center_axis',(0.,0.,-1.));
#20821=DIRECTION('ref_axis',(0.330288866442324,0.943879899512774,0.));
#20822=DIRECTION('center_axis',(-0.943879899512774,0.330288866442325,0.));
#20823=DIRECTION('ref_axis',(-0.330288866442325,-0.943879899512774,0.));
#20824=DIRECTION('center_axis',(0.,0.,1.));
#20825=DIRECTION('ref_axis',(0.330288866442325,0.943879899512774,0.));
#20826=DIRECTION('center_axis',(0.,0.,1.));
#20827=DIRECTION('ref_axis',(0.330288866442325,0.943879899512774,0.));
#20828=DIRECTION('center_axis',(0.,0.,1.));
#20829=DIRECTION('ref_axis',(-0.330288866442325,-0.943879899512774,0.));
#20830=DIRECTION('center_axis',(0.,0.,1.));
#20831=DIRECTION('ref_axis',(-0.330288866442324,-0.943879899512774,0.));
#20832=DIRECTION('center_axis',(-0.943879899512774,0.330288866442324,0.));
#20833=DIRECTION('ref_axis',(0.330288866442324,0.943879899512774,0.));
#20834=DIRECTION('center_axis',(0.,0.,-1.));
#20835=DIRECTION('ref_axis',(-0.330288866442325,-0.943879899512774,0.));
#20836=DIRECTION('center_axis',(0.,0.,1.));
#20837=DIRECTION('ref_axis',(-0.330288866442324,-0.943879899512774,0.));
#20838=DIRECTION('center_axis',(0.,0.,1.));
#20839=DIRECTION('ref_axis',(-0.330288866442324,-0.943879899512774,0.));
#20840=DIRECTION('center_axis',(0.943879899512774,-0.330288866442325,0.));
#20841=DIRECTION('ref_axis',(0.330288866442325,0.943879899512774,0.));
#20842=DIRECTION('center_axis',(0.,0.,-1.));
#20843=DIRECTION('ref_axis',(-0.330288866442325,-0.943879899512774,0.));
#20844=DIRECTION('center_axis',(0.,0.,1.));
#20845=DIRECTION('ref_axis',(-0.330288866442324,-0.943879899512774,0.));
#20846=DIRECTION('center_axis',(0.,0.,1.));
#20847=DIRECTION('ref_axis',(0.330288866442325,0.943879899512774,0.));
#20848=DIRECTION('center_axis',(-0.943879899512774,0.330288866442324,0.));
#20849=DIRECTION('ref_axis',(0.330288866442324,0.943879899512774,0.));
#20850=DIRECTION('center_axis',(0.,0.,-1.));
#20851=DIRECTION('ref_axis',(-0.330288866442325,-0.943879899512774,0.));
#20852=DIRECTION('center_axis',(0.,0.,1.));
#20853=DIRECTION('ref_axis',(-0.330288866442324,-0.943879899512774,0.));
#20854=DIRECTION('center_axis',(0.,0.,1.));
#20855=DIRECTION('ref_axis',(-0.330288866442325,-0.943879899512774,0.));
#20856=DIRECTION('center_axis',(-0.943879899512774,0.330288866442325,0.));
#20857=DIRECTION('ref_axis',(0.330288866442324,0.943879899512774,0.));
#20858=DIRECTION('center_axis',(0.,0.,-1.));
#20859=DIRECTION('ref_axis',(-0.330288866442324,-0.943879899512774,0.));
#20860=DIRECTION('center_axis',(0.,0.,1.));
#20861=DIRECTION('ref_axis',(-0.330288866442324,-0.943879899512774,0.));
#20862=DIRECTION('',(0.,0.,-1.));
#20863=DIRECTION('center_axis',(0.,0.,1.));
#20864=DIRECTION('ref_axis',(-0.330288866442325,-0.943879899512774,0.));
#20865=DIRECTION('',(0.,0.,-1.));
#20866=DIRECTION('center_axis',(0.,0.,-1.));
#20867=DIRECTION('ref_axis',(-1.,0.,0.));
#20868=DIRECTION('center_axis',(0.,0.,1.));
#20869=DIRECTION('ref_axis',(-0.330288866442325,-0.943879899512774,0.));
#20870=DIRECTION('center_axis',(0.,0.,-1.));
#20871=DIRECTION('ref_axis',(-1.,0.,0.));
#20872=DIRECTION('center_axis',(0.,0.,1.));
#20873=DIRECTION('ref_axis',(-0.330288866442325,-0.943879899512774,0.));
#20874=DIRECTION('center_axis',(0.,0.,-1.));
#20875=DIRECTION('ref_axis',(-1.,0.,0.));
#20876=DIRECTION('center_axis',(0.,0.,1.));
#20877=DIRECTION('ref_axis',(-0.330288866442325,-0.943879899512774,0.));
#20878=DIRECTION('center_axis',(0.,0.,-1.));
#20879=DIRECTION('ref_axis',(-1.,0.,0.));
#20880=DIRECTION('center_axis',(0.,0.,1.));
#20881=DIRECTION('ref_axis',(-0.330288866442325,-0.943879899512774,0.));
#20882=DIRECTION('center_axis',(0.,0.,-1.));
#20883=DIRECTION('ref_axis',(-1.,0.,0.));
#20884=DIRECTION('center_axis',(0.,0.,1.));
#20885=DIRECTION('ref_axis',(-0.330288866442325,-0.943879899512774,0.));
#20886=DIRECTION('center_axis',(0.,0.,-1.));
#20887=DIRECTION('ref_axis',(-1.,0.,0.));
#20888=DIRECTION('center_axis',(0.,0.,1.));
#20889=DIRECTION('ref_axis',(-0.330288866442324,-0.943879899512774,0.));
#20890=DIRECTION('center_axis',(0.,0.,-1.));
#20891=DIRECTION('ref_axis',(-1.,0.,0.));
#20892=DIRECTION('center_axis',(0.,0.,-1.));
#20893=DIRECTION('ref_axis',(-1.,0.,0.));
#20894=DIRECTION('center_axis',(0.,0.,-1.));
#20895=DIRECTION('ref_axis',(-1.,0.,0.));
#20896=DIRECTION('center_axis',(0.,0.,-1.));
#20897=DIRECTION('ref_axis',(-1.,0.,0.));
#20898=DIRECTION('',(-0.014665028342131,-0.0419088467226302,-0.999013806466209));
#20899=DIRECTION('center_axis',(0.,0.,-1.));
#20900=DIRECTION('ref_axis',(-1.,0.,0.));
#20901=DIRECTION('center_axis',(0.,0.,-1.));
#20902=DIRECTION('ref_axis',(-1.,0.,0.));
#20903=DIRECTION('center_axis',(0.,0.,-1.));
#20904=DIRECTION('ref_axis',(-1.,0.,0.));
#20905=DIRECTION('center_axis',(0.,0.,1.));
#20906=DIRECTION('ref_axis',(-0.330288866442325,-0.943879899512774,0.));
#20907=DIRECTION('center_axis',(0.,0.,1.));
#20908=DIRECTION('ref_axis',(-0.330288866442324,-0.943879899512774,0.));
#20909=DIRECTION('',(0.,0.,1.));
#20910=DIRECTION('center_axis',(0.,0.,1.));
#20911=DIRECTION('ref_axis',(-0.330288866442325,-0.943879899512774,0.));
#20912=DIRECTION('center_axis',(0.,0.,1.));
#20913=DIRECTION('ref_axis',(-0.330288866442325,-0.943879899512774,0.));
#20914=DIRECTION('',(0.,0.,1.));
#20915=DIRECTION('center_axis',(0.,0.,-1.));
#20916=DIRECTION('ref_axis',(0.943879899512774,-0.330288866442325,0.));
#20917=DIRECTION('center_axis',(0.,0.,1.));
#20918=DIRECTION('ref_axis',(-0.330288866442324,-0.943879899512774,0.));
#20919=DIRECTION('center_axis',(0.,0.,1.));
#20920=DIRECTION('ref_axis',(-0.330288866442324,-0.943879899512774,0.));
#20921=DIRECTION('',(0.,0.,-1.));
#20922=DIRECTION('center_axis',(0.,0.,-1.));
#20923=DIRECTION('ref_axis',(0.330288866442324,0.943879899512774,0.));
#20924=DIRECTION('',(0.330247702396689,0.94376226334878,0.0157875058352114));
#20925=DIRECTION('center_axis',(0.,0.,1.));
#20926=DIRECTION('ref_axis',(-0.330288866442325,-0.943879899512774,0.));
#20927=DIRECTION('center_axis',(0.,0.,1.));
#20928=DIRECTION('ref_axis',(-0.236333478439911,-0.971672005858197,0.));
#20929=DIRECTION('center_axis',(0.,0.,1.));
#20930=DIRECTION('ref_axis',(-0.236333478439911,-0.971672005858197,0.));
#20931=DIRECTION('center_axis',(0.,0.,1.));
#20932=DIRECTION('ref_axis',(-0.236333478439911,-0.971672005858197,0.));
#20933=DIRECTION('center_axis',(-0.971672005858197,0.236333478439911,0.));
#20934=DIRECTION('ref_axis',(0.236333478439911,0.971672005858197,0.));
#20935=DIRECTION('center_axis',(0.,0.,-1.));
#20936=DIRECTION('ref_axis',(-0.236333478439911,-0.971672005858197,0.));
#20937=DIRECTION('center_axis',(0.,0.,-1.));
#20938=DIRECTION('ref_axis',(0.236333478439911,0.971672005858197,0.));
#20939=DIRECTION('center_axis',(0.,0.,-1.));
#20940=DIRECTION('ref_axis',(0.236333478439911,0.971672005858197,0.));
#20941=DIRECTION('center_axis',(0.971672005858197,-0.236333478439911,0.));
#20942=DIRECTION('ref_axis',(-0.236333478439911,-0.971672005858197,0.));
#20943=DIRECTION('center_axis',(0.,0.,1.));
#20944=DIRECTION('ref_axis',(0.236333478439911,0.971672005858197,0.));
#20945=DIRECTION('center_axis',(0.,0.,1.));
#20946=DIRECTION('ref_axis',(-0.236333478439911,-0.971672005858197,0.));
#20947=DIRECTION('center_axis',(0.,0.,1.));
#20948=DIRECTION('ref_axis',(-0.236333478439911,-0.971672005858197,0.));
#20949=DIRECTION('center_axis',(0.,0.,1.));
#20950=DIRECTION('ref_axis',(-0.236333478439911,-0.971672005858197,0.));
#20951=DIRECTION('center_axis',(-0.971672005858197,0.236333478439911,0.));
#20952=DIRECTION('ref_axis',(0.236333478439911,0.971672005858197,0.));
#20953=DIRECTION('center_axis',(0.,0.,-1.));
#20954=DIRECTION('ref_axis',(0.236333478439911,0.971672005858197,0.));
#20955=DIRECTION('center_axis',(-0.525029657457558,-0.851083931695341,0.));
#20956=DIRECTION('ref_axis',(0.851083931695341,-0.525029657457558,0.));
#20957=DIRECTION('',(0.525029657457553,0.851083931695343,0.));
#20958=DIRECTION('center_axis',(0.525029657457559,0.85108393169534,2.96134752604748E-14));
#20959=DIRECTION('ref_axis',(0.85108393169534,-0.525029657457559,-7.40770614500254E-28));
#20960=DIRECTION('',(-0.525029657457553,-0.851083931695343,0.));
#20961=DIRECTION('center_axis',(0.,0.,1.));
#20962=DIRECTION('ref_axis',(1.,0.,0.));
#20963=DIRECTION('center_axis',(0.0200037109101317,0.0324264290370445,0.999273925532799));
#20964=DIRECTION('ref_axis',(-0.23617825252725,-0.971033803116402,0.0362379116185115));
#20965=DIRECTION('center_axis',(0.872062858341818,-0.489393881347834,0.));
#20966=DIRECTION('ref_axis',(0.489393881347834,0.872062858341818,0.));
#20967=DIRECTION('center_axis',(0.,0.,-1.));
#20968=DIRECTION('ref_axis',(0.236333478439912,0.971672005858197,0.));
#20969=DIRECTION('center_axis',(0.,0.,-1.));
#20970=DIRECTION('ref_axis',(0.236333478439911,0.971672005858197,0.));
#20971=DIRECTION('center_axis',(0.788606312050867,0.61489843437232,-2.04787185540381E-15));
#20972=DIRECTION('ref_axis',(0.61489843437232,-0.788606312050867,5.79335698387264E-29));
#20973=DIRECTION('center_axis',(-0.0200042106442368,-0.0324272391163663,
-0.999273889241479));
#20974=DIRECTION('ref_axis',(0.851083931702766,-0.525029657445522,-5.68435167261249E-13));
#20975=DIRECTION('',(0.0199847256250061,0.0324383169330875,0.999273919571727));
#20976=DIRECTION('',(-0.526267548714368,-0.850319038461532,-1.61440824337016E-7));
#20977=DIRECTION('',(-0.0200040683734365,-0.0324270084924563,-0.999273899573456));
#20978=DIRECTION('center_axis',(0.,0.,-1.));
#20979=DIRECTION('ref_axis',(0.236333478439934,0.971672005858191,0.));
#20980=DIRECTION('',(0.,0.,-1.));
#20981=DIRECTION('',(0.,0.,1.));
#20982=DIRECTION('center_axis',(0.,0.,-1.));
#20983=DIRECTION('ref_axis',(0.236333478439934,0.971672005858191,0.));
#20984=DIRECTION('center_axis',(0.,0.,-1.));
#20985=DIRECTION('ref_axis',(0.236333478439911,0.971672005858197,0.));
#20986=DIRECTION('center_axis',(0.,0.,1.));
#20987=DIRECTION('ref_axis',(0.236333478439915,0.971672005858196,0.));
#20988=DIRECTION('center_axis',(0.,0.,-1.));
#20989=DIRECTION('ref_axis',(0.236333478439911,0.971672005858197,0.));
#20990=DIRECTION('center_axis',(0.,0.,1.));
#20991=DIRECTION('ref_axis',(1.,0.,0.));
#20992=DIRECTION('center_axis',(-0.0246581606679246,0.0290453078379217,
0.999273908998466));
#20993=DIRECTION('ref_axis',(0.971210061729006,-0.236221122766167,0.0308317556333084));
#20994=DIRECTION('center_axis',(0.647185832447695,-0.762332275506543,0.));
#20995=DIRECTION('ref_axis',(0.762332275506543,0.647185832447695,0.));
#20996=DIRECTION('center_axis',(0.,0.,-1.));
#20997=DIRECTION('ref_axis',(0.236333478439911,0.971672005858197,0.));
#20998=DIRECTION('center_axis',(0.,0.,-1.));
#20999=DIRECTION('ref_axis',(0.236333478439911,0.971672005858197,0.));
#21000=DIRECTION('center_axis',(0.,0.,1.));
#21001=DIRECTION('ref_axis',(0.236333478439904,0.971672005858199,0.));
#21002=DIRECTION('center_axis',(0.,0.,-1.));
#21003=DIRECTION('ref_axis',(0.236333478439911,0.971672005858197,0.));
#21004=DIRECTION('center_axis',(0.,0.,-1.));
#21005=DIRECTION('ref_axis',(0.236333478439911,0.971672005858197,0.));
#21006=DIRECTION('center_axis',(0.,0.,1.));
#21007=DIRECTION('ref_axis',(0.23633347843988,0.971672005858205,0.));
#21008=DIRECTION('center_axis',(-0.647185832447714,0.762332275506527,0.));
#21009=DIRECTION('ref_axis',(-0.762332275506527,-0.647185832447714,0.));
#21010=DIRECTION('',(-0.647185832447714,0.762332275506527,0.));
#21011=DIRECTION('',(0.647185832447714,-0.762332275506527,0.));
#21012=DIRECTION('center_axis',(-0.0246584553606204,0.0290456549619493,
0.999273891636852));
#21013=DIRECTION('ref_axis',(-0.762332275500488,-0.647185832454827,4.26326374061232E-13));
#21014=DIRECTION('',(-0.0246586071825858,0.0290458337958772,0.999273882692286));
#21015=DIRECTION('',(-0.648187897113365,0.761480433127297,1.32007699339018E-7));
#21016=DIRECTION('',(0.0246410696828602,-0.0290600164161832,-0.99927390295693));
#21017=DIRECTION('center_axis',(0.0200039468311077,0.0324268114698234,0.999273908400034));
#21018=DIRECTION('ref_axis',(-0.851083931689181,0.525029657467544,-4.26326364282818E-13));
#21019=DIRECTION('',(-0.0200228534542546,-0.0324147960551628,-0.999273919571732));
#21020=DIRECTION('',(0.0200040683734419,0.0324270084924578,0.999273899573456));
#21021=DIRECTION('',(0.523790654476959,0.851847022817227,1.61489583376044E-7));
#21022=DIRECTION('center_axis',(0.,0.,-1.));
#21023=DIRECTION('ref_axis',(0.236333478439934,0.971672005858191,0.));
#21024=DIRECTION('center_axis',(0.,0.,-1.));
#21025=DIRECTION('ref_axis',(-0.236333478439934,-0.971672005858191,0.));
#21026=DIRECTION('',(0.,0.,1.));
#21027=DIRECTION('center_axis',(0.,0.,-1.));
#21028=DIRECTION('ref_axis',(0.236333478439934,0.971672005858191,0.));
#21029=DIRECTION('',(0.,0.,-1.));
#21030=DIRECTION('center_axis',(0.,0.,-1.));
#21031=DIRECTION('ref_axis',(0.236333478439934,0.971672005858191,0.));
#21032=DIRECTION('center_axis',(0.,0.,-1.));
#21033=DIRECTION('ref_axis',(0.236333478439934,0.971672005858191,0.));
#21034=DIRECTION('',(0.,0.,-1.));
#21035=DIRECTION('',(0.,0.,1.));
#21036=DIRECTION('center_axis',(0.,0.,-1.));
#21037=DIRECTION('ref_axis',(0.236333478439911,0.971672005858197,0.));
#21038=DIRECTION('center_axis',(0.,0.,1.));
#21039=DIRECTION('ref_axis',(0.236333478439911,0.971672005858197,0.));
#21040=DIRECTION('center_axis',(0.,0.,-1.));
#21041=DIRECTION('ref_axis',(0.236333478439911,0.971672005858197,0.));
#21042=DIRECTION('center_axis',(1.,0.,0.));
#21043=DIRECTION('ref_axis',(0.,-1.,0.));
#21044=DIRECTION('center_axis',(-0.82998202866415,0.557790132661507,0.));
#21045=DIRECTION('ref_axis',(-0.557790132661507,-0.82998202866415,0.));
#21046=DIRECTION('center_axis',(0.525029657457559,0.85108393169534,0.));
#21047=DIRECTION('ref_axis',(-0.85108393169534,0.525029657457559,0.));
#21048=DIRECTION('center_axis',(0.,0.,-1.));
#21049=DIRECTION('ref_axis',(0.236333478439911,0.971672005858197,0.));
#21050=DIRECTION('center_axis',(0.,0.,1.));
#21051=DIRECTION('ref_axis',(0.236333478439911,0.971672005858197,0.));
#21052=DIRECTION('center_axis',(0.,0.,-1.));
#21053=DIRECTION('ref_axis',(0.236333478439911,0.971672005858197,0.));
#21054=DIRECTION('center_axis',(0.0246582090638531,-0.0290453648443879,
-0.999273906147268));
#21055=DIRECTION('ref_axis',(0.762332275496643,0.647185832459356,-5.68435154081849E-13));
#21056=DIRECTION('',(-0.0246746594650707,0.0290303609984873,0.999273936075879));
#21057=DIRECTION('',(0.645969033808723,-0.763363614118585,-1.94028037441531E-7));
#21058=DIRECTION('',(0.0246580360155412,-0.0290451610075496,-0.999273916342212));
#21059=DIRECTION('center_axis',(0.,0.,-1.));
#21060=DIRECTION('ref_axis',(0.236333478439912,0.971672005858197,0.));
#21061=DIRECTION('center_axis',(0.19595899650011,0.980612090324543,0.));
#21062=DIRECTION('ref_axis',(0.980612090324543,-0.19595899650011,0.));
#21063=DIRECTION('center_axis',(0.,0.,-1.));
#21064=DIRECTION('ref_axis',(0.236333478439911,0.971672005858197,0.));
#21065=DIRECTION('center_axis',(0.525029657457558,0.851083931695341,0.));
#21066=DIRECTION('ref_axis',(-0.851083931695341,0.525029657457558,0.));
#21067=DIRECTION('',(-0.525029657457553,-0.851083931695343,0.));
#21068=DIRECTION('',(0.525029657457554,0.851083931695343,0.));
#21069=DIRECTION('center_axis',(0.,0.,-1.));
#21070=DIRECTION('ref_axis',(0.236333478439911,0.971672005858197,0.));
#21071=DIRECTION('center_axis',(0.,0.,-1.));
#21072=DIRECTION('ref_axis',(0.236333478439911,0.971672005858197,0.));
#21073=DIRECTION('center_axis',(0.,0.,1.));
#21074=DIRECTION('ref_axis',(0.236333478439915,0.971672005858196,0.));
#21075=DIRECTION('center_axis',(0.,0.,-1.));
#21076=DIRECTION('ref_axis',(0.236333478439934,0.971672005858191,0.));
#21077=DIRECTION('center_axis',(0.,0.,-1.));
#21078=DIRECTION('ref_axis',(-0.236333478439934,-0.971672005858191,0.));
#21079=DIRECTION('',(0.,0.,1.));
#21080=DIRECTION('center_axis',(0.,0.,-1.));
#21081=DIRECTION('ref_axis',(0.236333478439934,0.971672005858191,0.));
#21082=DIRECTION('',(0.,0.,-1.));
#21083=DIRECTION('center_axis',(0.,0.,1.));
#21084=DIRECTION('ref_axis',(-0.843255399479467,-0.537513098676418,0.));
#21085=DIRECTION('center_axis',(0.0370208532576562,-0.00900434197182349,
0.999273925532799));
#21086=DIRECTION('ref_axis',(0.970966499624253,-0.236161882735454,-0.0381001542027123));
#21087=DIRECTION('center_axis',(-0.971672005858197,0.236333478439911,-2.77555756156289E-14));
#21088=DIRECTION('ref_axis',(-2.6969315832187E-14,6.55957173134355E-15,
1.));
#21089=DIRECTION('center_axis',(1.,0.,0.));
#21090=DIRECTION('ref_axis',(0.,-1.,0.));
#21091=DIRECTION('center_axis',(-0.647185832447725,0.762332275506517,0.));
#21092=DIRECTION('ref_axis',(-0.762332275506517,-0.647185832447725,0.));
#21093=DIRECTION('center_axis',(0.736713387417931,0.676205135147019,-7.7165199669874E-15));
#21094=DIRECTION('ref_axis',(-0.676205135147019,0.736713387417931,-1.538061318188E-28));
#21095=DIRECTION('center_axis',(0.647185832447714,-0.762332275506527,0.));
#21096=DIRECTION('ref_axis',(0.762332275506527,0.647185832447714,0.));
#21097=DIRECTION('',(-0.647185832447714,0.762332275506527,0.));
#21098=DIRECTION('',(0.647185832447714,-0.762332275506527,0.));
#21099=DIRECTION('center_axis',(0.,0.,-1.));
#21100=DIRECTION('ref_axis',(0.236333478439912,0.971672005858197,0.));
#21101=DIRECTION('center_axis',(0.,0.,-1.));
#21102=DIRECTION('ref_axis',(0.236333478439911,0.971672005858197,0.));
#21103=DIRECTION('center_axis',(-0.037021778116286,0.00900456691918861,
-0.999273889241436));
#21104=DIRECTION('ref_axis',(-0.236333478439919,-0.971672005858195,0.));
#21105=DIRECTION('',(0.0370262925428981,-0.00898261233079703,0.999273919571727));
#21106=DIRECTION('',(-0.971327078599407,0.237747147994493,-1.61440824441445E-7));
#21107=DIRECTION('',(-0.0370215148147375,0.00900450287806102,-0.999273899573456));
#21108=DIRECTION('center_axis',(-0.971672005858197,0.236333478439911,0.));
#21109=DIRECTION('ref_axis',(-0.236333478439911,-0.971672005858197,0.));
#21110=DIRECTION('',(-0.971672005858197,0.236333478439911,0.));
#21111=DIRECTION('',(0.971672005858197,-0.236333478439911,0.));
#21112=DIRECTION('center_axis',(0.,0.,-1.));
#21113=DIRECTION('ref_axis',(0.236333478439934,0.971672005858191,0.));
#21114=DIRECTION('',(0.,0.,-1.));
#21115=DIRECTION('',(0.,0.,1.));
#21116=DIRECTION('center_axis',(0.,0.,-1.));
#21117=DIRECTION('ref_axis',(0.236333478439934,0.971672005858191,0.));
#21118=DIRECTION('center_axis',(0.,0.,-1.));
#21119=DIRECTION('ref_axis',(0.236333478439911,0.971672005858197,0.));
#21120=DIRECTION('center_axis',(-0.34321561568671,0.939256642855824,0.));
#21121=DIRECTION('ref_axis',(0.939256642855824,0.34321561568671,0.));
#21122=DIRECTION('center_axis',(0.,0.,1.));
#21123=DIRECTION('ref_axis',(0.236333478439911,0.971672005858197,0.));
#21124=DIRECTION('center_axis',(0.,0.,-1.));
#21125=DIRECTION('ref_axis',(0.236333478439911,0.971672005858197,0.));
#21126=DIRECTION('center_axis',(0.,0.,-1.));
#21127=DIRECTION('ref_axis',(0.236333478439911,0.971672005858197,0.));
#21128=DIRECTION('center_axis',(0.,0.,-1.));
#21129=DIRECTION('ref_axis',(0.236333478439911,0.971672005858197,0.));
#21130=DIRECTION('center_axis',(0.,0.,1.));
#21131=DIRECTION('ref_axis',(0.236333478439911,0.971672005858197,0.));
#21132=DIRECTION('center_axis',(0.,0.,-1.));
#21133=DIRECTION('ref_axis',(0.236333478439911,0.971672005858197,0.));
#21134=DIRECTION('center_axis',(0.,0.,-1.));
#21135=DIRECTION('ref_axis',(0.236333478439911,0.971672005858197,0.));
#21136=DIRECTION('center_axis',(0.,0.,1.));
#21137=DIRECTION('ref_axis',(0.236333478439891,0.971672005858202,0.));
#21138=DIRECTION('center_axis',(1.,0.,0.));
#21139=DIRECTION('ref_axis',(0.,-1.,0.));
#21140=DIRECTION('center_axis',(0.,0.,1.));
#21141=DIRECTION('ref_axis',(-0.236333478439908,-0.971672005858198,0.));
#21142=DIRECTION('center_axis',(-0.925012498947636,-0.37993667471126,4.07857950393881E-15));
#21143=DIRECTION('ref_axis',(0.37993667471126,-0.925012498947636,-5.72282343898698E-29));
#21144=DIRECTION('center_axis',(-0.925012498947636,-0.37993667471126,0.));
#21145=DIRECTION('ref_axis',(0.37993667471126,-0.925012498947636,0.));
#21146=DIRECTION('',(-0.925012498947635,-0.379936674711261,0.));
#21147=DIRECTION('',(0.925012498947635,0.379936674711261,0.));
#21148=DIRECTION('center_axis',(-0.0352441938793423,-0.0144760874481498,
0.999273881220754));
#21149=DIRECTION('ref_axis',(0.379936674734162,-0.925012498938229,9.94761553655057E-13));
#21150=DIRECTION('',(-0.0352444126515999,-0.0144761773059668,0.999273872202936));
#21151=DIRECTION('',(-0.924544964574144,-0.381072970020941,1.15083568972965E-7));
#21152=DIRECTION('',(0.0352525125757934,0.0144550288485472,-0.999273892633087));
#21153=DIRECTION('center_axis',(0.0370212898762763,-0.0090044481677379,
0.99927390840004));
#21154=DIRECTION('ref_axis',(0.236333478441325,0.971672005857853,0.));
#21155=DIRECTION('',(-0.0370157050058834,0.00902614240225516,-0.999273919571732));
#21156=DIRECTION('center_axis',(-0.0370208532576561,0.009004341971824,-0.999273925532799));
#21157=DIRECTION('ref_axis',(0.970966499624253,-0.236161882735454,-0.0381001542027123));
#21158=DIRECTION('',(0.0370215148147411,-0.00900450287806193,0.999273899573456));
#21159=DIRECTION('',(0.972014875666751,-0.234919308449784,1.61392065502938E-7));
#21160=DIRECTION('center_axis',(0.,0.,-1.));
#21161=DIRECTION('ref_axis',(0.236333478439934,0.971672005858191,0.));
#21162=DIRECTION('',(0.,0.,1.));
#21163=DIRECTION('center_axis',(0.,0.,-1.));
#21164=DIRECTION('ref_axis',(0.236333478439934,0.971672005858191,0.));
#21165=DIRECTION('',(0.,0.,-1.));
#21166=DIRECTION('center_axis',(0.,0.,-1.));
#21167=DIRECTION('ref_axis',(-0.403523989416176,-0.914969065032066,0.));
#21168=DIRECTION('center_axis',(0.,0.,-1.));
#21169=DIRECTION('ref_axis',(0.236333478439908,0.971672005858198,0.));
#21170=DIRECTION('',(0.,0.,-1.));
#21171=DIRECTION('',(0.,0.,1.));
#21172=DIRECTION('center_axis',(0.,0.,-1.));
#21173=DIRECTION('ref_axis',(0.236333478439911,0.971672005858197,0.));
#21174=DIRECTION('center_axis',(0.,0.,1.));
#21175=DIRECTION('ref_axis',(0.236333478439923,0.971672005858194,0.));
#21176=DIRECTION('center_axis',(0.,0.,-1.));
#21177=DIRECTION('ref_axis',(0.236333478439911,0.971672005858197,0.));
#21178=DIRECTION('center_axis',(-0.23633347843992,-0.971672005858195,0.));
#21179=DIRECTION('ref_axis',(0.,0.,1.));
#21180=DIRECTION('center_axis',(0.276303824482695,0.961070339036762,1.44037777350484E-15));
#21181=DIRECTION('ref_axis',(-0.961070339036762,0.276303824482695,1.44348006936188E-29));
#21182=DIRECTION('center_axis',(-0.97167200585819,0.236333478439938,0.));
#21183=DIRECTION('ref_axis',(-0.236333478439938,-0.97167200585819,0.));
#21184=DIRECTION('center_axis',(0.,0.,-1.));
#21185=DIRECTION('ref_axis',(0.236333478439911,0.971672005858197,0.));
#21186=DIRECTION('center_axis',(0.,0.,1.));
#21187=DIRECTION('ref_axis',(0.236333478439911,0.971672005858197,0.));
#21188=DIRECTION('center_axis',(0.,0.,-1.));
#21189=DIRECTION('ref_axis',(0.236333478439911,0.971672005858197,0.));
#21190=DIRECTION('center_axis',(0.0352433370446482,0.0144757355146047,-0.999273916539038));
#21191=DIRECTION('ref_axis',(-0.379936674702656,0.92501249895117,2.84217572986559E-13));
#21192=DIRECTION('center_axis',(0.0352424754478559,0.0144753816250977,-0.999273952052747));
#21193=DIRECTION('ref_axis',(0.97121008913075,-0.23622112943089,0.0308308413935825));
#21194=DIRECTION('',(-0.0352341919267929,-0.0144959347334989,0.999273946220689));
#21195=DIRECTION('',(0.925650075050678,0.378380679420379,-2.15610283786586E-7));
#21196=DIRECTION('',(0.0352430917530489,0.0144756347643183,-0.999273926649673));
#21197=DIRECTION('center_axis',(0.,0.,-1.));
#21198=DIRECTION('ref_axis',(0.236333478439912,0.971672005858197,0.));
#21199=DIRECTION('center_axis',(0.,0.,-1.));
#21200=DIRECTION('ref_axis',(0.236333478439911,0.971672005858197,0.));
#21201=DIRECTION('center_axis',(0.971672005858197,-0.236333478439911,0.));
#21202=DIRECTION('ref_axis',(0.236333478439911,0.971672005858197,0.));
#21203=DIRECTION('',(-0.971672005858197,0.236333478439911,0.));
#21204=DIRECTION('',(0.971672005858197,-0.236333478439911,0.));
#21205=DIRECTION('center_axis',(0.,0.,-1.));
#21206=DIRECTION('ref_axis',(0.236333478439911,0.971672005858197,0.));
#21207=DIRECTION('center_axis',(0.993477056368512,0.114032181726723,-4.79607696935732E-15));
#21208=DIRECTION('ref_axis',(0.114032181726723,-0.993477056368512,3.69174078276775E-29));
#21209=DIRECTION('center_axis',(0.,0.,-1.));
#21210=DIRECTION('ref_axis',(0.236333478439911,0.971672005858197,0.));
#21211=DIRECTION('center_axis',(0.,0.,1.));
#21212=DIRECTION('ref_axis',(0.236333478439912,0.971672005858197,0.));
#21213=DIRECTION('center_axis',(0.,0.,-1.));
#21214=DIRECTION('ref_axis',(0.236333478439908,0.971672005858198,0.));
#21215=DIRECTION('',(0.,0.,1.));
#21216=DIRECTION('center_axis',(0.,0.,-1.));
#21217=DIRECTION('ref_axis',(0.236333478439908,0.971672005858198,0.));
#21218=DIRECTION('',(0.,0.,-1.));
#21219=DIRECTION('center_axis',(0.,0.,1.));
#21220=DIRECTION('ref_axis',(1.,0.,0.));
#21221=DIRECTION('center_axis',(-0.41745153963428,0.908699186781285,0.));
#21222=DIRECTION('ref_axis',(-0.908699186781285,-0.41745153963428,0.));
#21223=DIRECTION('center_axis',(0.925012498947636,0.37993667471126,-2.49982082791546E-14));
#21224=DIRECTION('ref_axis',(-0.37993667471126,0.925012498947636,3.50802986436712E-28));
#21225=DIRECTION('center_axis',(1.,0.,0.));
#21226=DIRECTION('ref_axis',(0.,-1.,0.));
#21227=DIRECTION('center_axis',(0.,0.,1.));
#21228=DIRECTION('ref_axis',(-0.236333478439928,-0.971672005858193,0.));
#21229=DIRECTION('center_axis',(0.0754966680795893,-0.997146054050699,0.));
#21230=DIRECTION('ref_axis',(0.997146054050699,0.0754966680795893,0.));
#21231=DIRECTION('center_axis',(0.925012498947636,0.37993667471126,0.));
#21232=DIRECTION('ref_axis',(-0.37993667471126,0.925012498947636,0.));
#21233=DIRECTION('',(-0.925012498947636,-0.379936674711261,0.));
#21234=DIRECTION('',(0.925012498947636,0.379936674711261,0.));
#21235=DIRECTION('center_axis',(0.,0.,-1.));
#21236=DIRECTION('ref_axis',(-0.525335493488004,-0.850895187012898,0.));
#21237=DIRECTION('center_axis',(0.,0.,-1.));
#21238=DIRECTION('ref_axis',(0.236333478439911,0.971672005858197,0.));
#21239=DIRECTION('center_axis',(-0.99942413970229,-0.0339321231333568,-6.28874166431797E-15));
#21240=DIRECTION('ref_axis',(-0.0339321231333568,0.99942413970229,-3.82846242175198E-29));
#21241=DIRECTION('center_axis',(-0.00287647308046481,0.0379919254018759,
-0.999273906147296));
#21242=DIRECTION('ref_axis',(-0.997146054050261,-0.0754966680853753,-2.84217577056821E-13));
#21243=DIRECTION('',(0.00289860077403835,-0.0379894563395136,0.99927393607588));
#21244=DIRECTION('',(-0.0739060517243553,0.997265208216189,-1.94028037262086E-7));
#21245=DIRECTION('',(-0.0028764528937826,0.0379916587798979,-0.999273916342212));
#21246=DIRECTION('center_axis',(-0.0754966680796036,0.997146054050698,0.));
#21247=DIRECTION('ref_axis',(-0.997146054050698,-0.0754966680796036,0.));
#21248=DIRECTION('',(-0.0754966680795988,0.997146054050699,0.));
#21249=DIRECTION('',(0.0754966680795988,-0.997146054050699,0.));
#21250=DIRECTION('center_axis',(0.,0.,-1.));
#21251=DIRECTION('ref_axis',(-0.636902289361219,-0.770944533547283,0.));
#21252=DIRECTION('',(0.,0.,-1.));
#21253=DIRECTION('',(0.,0.,1.));
#21254=DIRECTION('center_axis',(0.,0.,-1.));
#21255=DIRECTION('ref_axis',(0.236333478439928,0.971672005858193,0.));
#21256=DIRECTION('center_axis',(0.,0.,-1.));
#21257=DIRECTION('ref_axis',(-0.525317843056466,-0.850906083987242,0.));
#21258=DIRECTION('center_axis',(0.,0.,1.));
#21259=DIRECTION('ref_axis',(0.236333478439911,0.971672005858197,0.));
#21260=DIRECTION('center_axis',(0.,0.,-1.));
#21261=DIRECTION('ref_axis',(0.236333478439911,0.971672005858197,0.));
#21262=DIRECTION('center_axis',(0.,0.,-1.));
#21263=DIRECTION('ref_axis',(0.236333478439911,0.971672005858197,0.));
#21264=DIRECTION('center_axis',(0.,0.,1.));
#21265=DIRECTION('ref_axis',(1.,0.,0.));
#21266=DIRECTION('center_axis',(-0.0754966680795893,0.997146054050699,0.));
#21267=DIRECTION('ref_axis',(-0.997146054050699,-0.0754966680795893,0.));
#21268=DIRECTION('center_axis',(0.00287646743495555,-0.0379918508369929,
0.999273908998466));
#21269=DIRECTION('ref_axis',(-0.236178248992025,-0.971033788581598,-0.036238324132465));
#21270=DIRECTION('center_axis',(0.,0.,-1.));
#21271=DIRECTION('ref_axis',(0.236333478439911,0.971672005858197,0.));
#21272=DIRECTION('center_axis',(0.,0.,-1.));
#21273=DIRECTION('ref_axis',(0.236333478439911,0.971672005858197,0.));
#21274=DIRECTION('center_axis',(0.,0.,1.));
#21275=DIRECTION('ref_axis',(0.236333478439911,0.971672005858197,0.));
#21276=DIRECTION('center_axis',(0.,0.,-1.));
#21277=DIRECTION('ref_axis',(0.236333478439911,0.971672005858197,0.));
#21278=DIRECTION('center_axis',(0.,0.,-1.));
#21279=DIRECTION('ref_axis',(0.236333478439911,0.971672005858197,0.));
#21280=DIRECTION('center_axis',(0.,0.,1.));
#21281=DIRECTION('ref_axis',(0.236333478439911,0.971672005858197,0.));
#21282=DIRECTION('center_axis',(0.0754966680796036,-0.997146054050698,0.));
#21283=DIRECTION('ref_axis',(0.997146054050698,0.0754966680796036,0.));
#21284=DIRECTION('',(0.0754966680795988,-0.997146054050699,0.));
#21285=DIRECTION('',(-0.0754966680795988,0.997146054050699,0.));
#21286=DIRECTION('center_axis',(0.00287650181214345,-0.0379923048845794,
0.999273891636763));
#21287=DIRECTION('ref_axis',(0.997146054051204,0.0754966680729282,-2.84217582707585E-13));
#21288=DIRECTION('',(-0.00285399505219986,0.0379937044978036,-0.99927390295693));
#21289=DIRECTION('',(0.0028765195225703,-0.0379925388006534,0.999273882692286));
#21290=DIRECTION('',(0.0768080558201112,-0.997045897921012,1.31953752638336E-7));
#21291=DIRECTION('center_axis',(0.,0.,-1.));
#21292=DIRECTION('ref_axis',(0.236333478439928,0.971672005858193,0.));
#21293=DIRECTION('center_axis',(0.,0.,-1.));
#21294=DIRECTION('ref_axis',(0.236333478439928,0.971672005858193,0.));
#21295=DIRECTION('',(0.,0.,-1.));
#21296=DIRECTION('',(0.,0.,1.));
#21297=DIRECTION('center_axis',(0.,0.,-1.));
#21298=DIRECTION('ref_axis',(0.236333478439911,0.971672005858197,0.));
#21299=DIRECTION('center_axis',(0.,0.,-1.));
#21300=DIRECTION('ref_axis',(0.236333478439911,0.971672005858197,0.));
#21301=DIRECTION('center_axis',(-0.971672005858197,0.236333478439911,0.));
#21302=DIRECTION('ref_axis',(-0.236333478439911,-0.971672005858197,0.));
#21303=DIRECTION('center_axis',(0.,0.,1.));
#21304=DIRECTION('ref_axis',(0.236333478439911,0.971672005858197,0.));
#21305=DIRECTION('center_axis',(0.,0.,-1.));
#21306=DIRECTION('ref_axis',(0.236333478439911,0.971672005858197,0.));
#21307=DIRECTION('',(-0.971672005858197,0.236333478439911,0.));
#21308=DIRECTION('',(0.971672005858197,-0.236333478439911,0.));
#21309=DIRECTION('center_axis',(-0.236333478439911,-0.971672005858197,0.));
#21310=DIRECTION('ref_axis',(0.,0.,-1.));
#21311=DIRECTION('center_axis',(0.236333478439911,0.971672005858197,0.));
#21312=DIRECTION('ref_axis',(-0.971672005858197,0.236333478439911,0.));
#21313=DIRECTION('center_axis',(0.,0.,-1.));
#21314=DIRECTION('ref_axis',(0.236333478439911,0.971672005858197,0.));
#21315=DIRECTION('',(-0.0754966680795988,0.997146054050699,0.));
#21316=DIRECTION('',(0.0754966680795988,-0.997146054050699,0.));
#21317=DIRECTION('center_axis',(0.997146054050699,0.0754966680795988,0.));
#21318=DIRECTION('ref_axis',(0.,0.,1.));
#21319=DIRECTION('center_axis',(-0.997146054050699,-0.0754966680795988,
0.));
#21320=DIRECTION('ref_axis',(0.0754966680795988,-0.997146054050699,0.));
#21321=DIRECTION('center_axis',(0.,0.,-1.));
#21322=DIRECTION('ref_axis',(0.236333478439911,0.971672005858197,0.));
#21323=DIRECTION('',(0.925012498947636,0.379936674711261,0.));
#21324=DIRECTION('',(-0.925012498947635,-0.379936674711261,0.));
#21325=DIRECTION('center_axis',(0.379936674711261,-0.925012498947636,0.));
#21326=DIRECTION('ref_axis',(0.,0.,-1.));
#21327=DIRECTION('center_axis',(-0.379936674711261,0.925012498947635,0.));
#21328=DIRECTION('ref_axis',(0.,0.,-1.));
#21329=DIRECTION('center_axis',(0.,0.,-1.));
#21330=DIRECTION('ref_axis',(0.236333478439911,0.971672005858197,0.));
#21331=DIRECTION('',(0.647185832447714,-0.762332275506527,0.));
#21332=DIRECTION('',(-0.647185832447714,0.762332275506527,0.));
#21333=DIRECTION('center_axis',(-0.762332275506527,-0.647185832447714,0.));
#21334=DIRECTION('ref_axis',(-0.647185832447714,0.762332275506527,0.));
#21335=DIRECTION('center_axis',(0.762332275506527,0.647185832447714,0.));
#21336=DIRECTION('ref_axis',(0.,0.,1.));
#21337=DIRECTION('center_axis',(0.,0.,-1.));
#21338=DIRECTION('ref_axis',(0.236333478439911,0.971672005858197,0.));
#21339=DIRECTION('',(-0.525029657457553,-0.851083931695343,0.));
#21340=DIRECTION('',(0.525029657457553,0.851083931695343,0.));
#21341=DIRECTION('center_axis',(-0.851083931695343,0.525029657457553,0.));
#21342=DIRECTION('ref_axis',(0.,0.,-1.));
#21343=DIRECTION('center_axis',(0.851083931695343,-0.525029657457553,0.));
#21344=DIRECTION('ref_axis',(0.,0.,-1.));
#21345=DIRECTION('center_axis',(0.,0.,1.));
#21346=DIRECTION('ref_axis',(0.971672005858197,-0.236333478439911,0.));
#21347=DIRECTION('center_axis',(0.,0.,-1.));
#21348=DIRECTION('ref_axis',(0.236333478439911,0.971672005858197,0.));
#21349=DIRECTION('center_axis',(0.,0.,-1.));
#21350=DIRECTION('ref_axis',(0.236333478439911,0.971672005858197,0.));
#21351=DIRECTION('center_axis',(0.,0.,-1.));
#21352=DIRECTION('ref_axis',(0.236333478439911,0.971672005858197,0.));
#21353=DIRECTION('center_axis',(-0.971672005858197,0.236333478439911,0.));
#21354=DIRECTION('ref_axis',(-0.236333478439911,-0.971672005858197,0.));
#21355=DIRECTION('center_axis',(0.,0.,-1.));
#21356=DIRECTION('ref_axis',(0.236333478439911,0.971672005858197,0.));
#21357=DIRECTION('',(0.,0.,-1.));
#21358=DIRECTION('center_axis',(0.,0.,1.));
#21359=DIRECTION('ref_axis',(-0.236333478439911,-0.971672005858197,0.));
#21360=DIRECTION('',(0.00899665431329341,0.0369892458754347,0.999275165257665));
#21361=DIRECTION('center_axis',(0.,0.,-1.));
#21362=DIRECTION('ref_axis',(0.236333478439911,0.971672005858197,0.));
#21363=DIRECTION('center_axis',(0.,0.,-1.));
#21364=DIRECTION('ref_axis',(0.236333478439911,0.971672005858197,0.));
#21365=DIRECTION('',(0.,0.,1.));
#21366=DIRECTION('center_axis',(0.,0.,-1.));
#21367=DIRECTION('ref_axis',(0.236333478439911,0.971672005858197,0.));
#21368=DIRECTION('center_axis',(0.,0.,-1.));
#21369=DIRECTION('ref_axis',(0.236333478439911,0.971672005858197,0.));
#21370=DIRECTION('',(0.,0.,1.));
#21371=DIRECTION('center_axis',(0.,0.,-1.));
#21372=DIRECTION('ref_axis',(0.236333478439911,0.971672005858197,0.));
#21373=DIRECTION('center_axis',(0.,0.,-1.));
#21374=DIRECTION('ref_axis',(0.236333478439911,0.971672005858197,0.));
#21375=DIRECTION('center_axis',(0.,0.,-1.));
#21376=DIRECTION('ref_axis',(0.236333478439911,0.971672005858197,0.));
#21377=DIRECTION('center_axis',(0.,0.,-1.));
#21378=DIRECTION('ref_axis',(0.236333478439911,0.971672005858197,0.));
#25558=CARTESIAN_POINT('',(0.,0.,0.));
#25559=CARTESIAN_POINT('Origin',(77.9152339218055,61.1315783931225,207.276481344607));
#25560=CARTESIAN_POINT('',(78.1645204353182,61.1504525601425,207.276481344607));
#25561=CARTESIAN_POINT('',(77.9152339218055,61.1315783931225,207.526481344607));
#25562=CARTESIAN_POINT('Origin',(77.9152339218055,61.1315783931226,207.276481344607));
#25563=CARTESIAN_POINT('',(77.9243166636283,60.8817434400015,207.276481344607));
#25564=CARTESIAN_POINT('Origin',(77.9152339218055,61.1315783931225,207.276481344607));
#25565=CARTESIAN_POINT('Origin',(77.9152339218055,61.1315783931226,207.276481344607));
#25566=CARTESIAN_POINT('Origin',(59.7044966368782,72.3742118764312,207.276481344607));
#25567=CARTESIAN_POINT('',(59.4770762970785,72.2703851503661,207.276481344607));
#25568=CARTESIAN_POINT('',(59.6095124682004,72.6054650011681,207.276481344607));
#25569=CARTESIAN_POINT('Origin',(59.7044966368782,72.3742118764312,207.276481344607));
#25570=CARTESIAN_POINT('',(59.7044966368782,72.3742118764312,207.526481344607));
#25571=CARTESIAN_POINT('Origin',(59.7044966368782,72.3742118764312,207.276481344607));
#25572=CARTESIAN_POINT('Origin',(59.7044966368782,72.3742118764312,207.276481344607));
#25573=CARTESIAN_POINT('Origin',(79.3271639989382,62.3514930904775,207.276481344607));
#25574=CARTESIAN_POINT('',(79.2329453452574,62.5828815339371,207.285549615221));
#25575=CARTESIAN_POINT('',(79.0778774854255,62.3326189234576,207.276481344607));
#25576=CARTESIAN_POINT('Origin',(79.3271639989382,62.3514930904775,207.276481344607));
#25577=CARTESIAN_POINT('',(79.3271639989382,62.3514930904775,207.526481344607));
#25578=CARTESIAN_POINT('Origin',(79.3271639989382,62.3514930904775,207.276481344607));
#25579=CARTESIAN_POINT('',(79.2991550620136,62.5905151532426,207.3441862409));
#25580=CARTESIAN_POINT('Origin',(79.3271639989382,62.3514930904775,207.276481344607));
#25581=CARTESIAN_POINT('Ctrl Pts',(79.2991550620136,62.5905151532426,207.344186240766));
#25582=CARTESIAN_POINT('Ctrl Pts',(79.2936414483863,62.5898690603484,207.344186240766));
#25583=CARTESIAN_POINT('Ctrl Pts',(79.2876554089815,62.5891704418728,207.343449242348));
#25584=CARTESIAN_POINT('Ctrl Pts',(79.2761242753789,62.5878305349169,207.340322634924));
#25585=CARTESIAN_POINT('Ctrl Pts',(79.2705791816217,62.5871892200478,207.337933035602));
#25586=CARTESIAN_POINT('Ctrl Pts',(79.260853293221,62.5860680140522,207.332255389429));
#25587=CARTESIAN_POINT('Ctrl Pts',(79.2561763647588,62.5855310114079,207.328654585832));
#25588=CARTESIAN_POINT('Ctrl Pts',(79.2478683053229,62.5845797700644,207.320274409274));
#25589=CARTESIAN_POINT('Ctrl Pts',(79.2442358923008,62.5841654166262,207.315496320451));
#25590=CARTESIAN_POINT('Ctrl Pts',(79.2369361747333,62.5833339506126,207.302683579489));
#25591=CARTESIAN_POINT('Ctrl Pts',(79.2340922950462,62.5830116078114,207.294147337792));
#25592=CARTESIAN_POINT('Ctrl Pts',(79.232945345238,62.582881533935,207.285549615073));
#25593=CARTESIAN_POINT('Origin',(95.7290969072821,75.0941505546249,207.276481344607));
#25594=CARTESIAN_POINT('',(95.788180276892,75.3370685560895,207.276481344607));
#25595=CARTESIAN_POINT('',(95.7290969072821,75.0941505546249,207.526481344607));
#25596=CARTESIAN_POINT('Origin',(95.7290969072821,75.0941505546249,207.276481344607));
#25597=CARTESIAN_POINT('',(95.969528519046,75.0256477074975,207.276481344607));
#25598=CARTESIAN_POINT('Origin',(95.7290969072821,75.0941505546249,207.276481344607));
#25599=CARTESIAN_POINT('Origin',(95.7290969072821,75.0941505546249,207.276481344607));
#25600=CARTESIAN_POINT('Origin',(60.1621734217283,74.1837962848936,207.276481344607));
#25601=CARTESIAN_POINT('',(60.1621734217283,74.1837962848936,207.526481344607));
#25602=CARTESIAN_POINT('',(60.3884110190581,74.2658486863688,207.344186240786));
#25603=CARTESIAN_POINT('Origin',(60.1621734217283,74.1837962848936,207.276481344607));
#25604=CARTESIAN_POINT('',(60.2571575904061,73.9525431601567,207.276481344607));
#25605=CARTESIAN_POINT('Origin',(60.1621734217283,74.1837962848936,207.276481344607));
#25606=CARTESIAN_POINT('',(60.4112511369769,74.2032374366335,207.285547783929));
#25607=CARTESIAN_POINT('Origin',(60.1621734217283,74.1837962848936,207.276481344607));
#25608=CARTESIAN_POINT('Ctrl Pts',(60.4112515042303,74.2032360650638,207.285547973752));
#25609=CARTESIAN_POINT('Ctrl Pts',(60.4108539539671,74.2043195996929,207.294146250025));
#25610=CARTESIAN_POINT('Ctrl Pts',(60.4098679175592,74.2070065582381,207.302683093175));
#25611=CARTESIAN_POINT('Ctrl Pts',(60.407340557639,74.2139053814473,207.315496320451));
#25612=CARTESIAN_POINT('Ctrl Pts',(60.4060835087816,74.2173384473227,207.320274409274));
#25613=CARTESIAN_POINT('Ctrl Pts',(60.4032115424655,74.2251921420687,207.328654585832));
#25614=CARTESIAN_POINT('Ctrl Pts',(60.4015961531691,74.2296139685129,207.332255389429));
#25615=CARTESIAN_POINT('Ctrl Pts',(60.3982408855922,74.2388113696434,207.337933035602));
#25616=CARTESIAN_POINT('Ctrl Pts',(60.3963297752376,74.2440560819091,207.340322634924));
#25617=CARTESIAN_POINT('Ctrl Pts',(60.3923611971915,74.254965379829,207.343449242348));
#25618=CARTESIAN_POINT('Ctrl Pts',(60.3903037532893,74.2606299769125,207.344186240766));
#25619=CARTESIAN_POINT('Ctrl Pts',(60.3884110190634,74.2658486863707,207.344186240766));
#25620=CARTESIAN_POINT('Origin',(96.0835971249419,76.5516585634122,207.276481344607));
#25621=CARTESIAN_POINT('',(96.0835971249419,76.5516585634122,207.526481344607));
#25622=CARTESIAN_POINT('',(96.3286326356366,76.5020843917236,207.276481344607));
#25623=CARTESIAN_POINT('Origin',(96.0835971249419,76.5516585634122,207.276481344607));
#25624=CARTESIAN_POINT('',(96.0245137553319,76.3087405619477,207.276481344607));
#25625=CARTESIAN_POINT('Origin',(96.0835971249419,76.5516585634122,207.276481344607));
#25626=CARTESIAN_POINT('Origin',(96.0835971249419,76.5516585634122,207.276481344607));
#25627=CARTESIAN_POINT('Origin',(64.9174359473229,93.7042420150737,207.276481344607));
#25628=CARTESIAN_POINT('',(65.1080190161996,93.8660384731857,207.276481344607));
#25629=CARTESIAN_POINT('',(64.9174359473229,93.7042420150737,207.526481344607));
#25630=CARTESIAN_POINT('Origin',(64.9174359473229,93.7042420150737,207.276481344607));
#25631=CARTESIAN_POINT('',(65.0805892967552,93.5273323443229,207.344186240766));
#25632=CARTESIAN_POINT('Origin',(64.9174359473229,93.7042420150737,207.276481344607));
#25633=CARTESIAN_POINT('',(65.1296671539667,93.5724251671486,207.285549615094));
#25634=CARTESIAN_POINT('Ctrl Pts',(65.0805892967552,93.5273323443229,207.344186240766));
#25635=CARTESIAN_POINT('Ctrl Pts',(65.0846701400053,93.5310958652313,207.344186240766));
#25636=CARTESIAN_POINT('Ctrl Pts',(65.0891023099758,93.5351795651324,207.343449242348));
#25637=CARTESIAN_POINT('Ctrl Pts',(65.0976436154766,93.5430414029044,207.340322634924));
#25638=CARTESIAN_POINT('Ctrl Pts',(65.1017527351394,93.5468195618653,207.337933035602));
#25639=CARTESIAN_POINT('Ctrl Pts',(65.108962115792,93.5534433703373,207.332255389428));
#25640=CARTESIAN_POINT('Ctrl Pts',(65.1124301881646,93.5566268441787,207.328654585832));
#25641=CARTESIAN_POINT('Ctrl Pts',(65.1185924238054,93.5622797694029,207.320274409274));
#25642=CARTESIAN_POINT('Ctrl Pts',(65.1212875568307,93.5647500671807,207.315496320451));
#25643=CARTESIAN_POINT('Ctrl Pts',(65.1267044289337,93.5697134036456,207.302683579495));
#25644=CARTESIAN_POINT('Ctrl Pts',(65.128815707585,93.5716457749885,207.294147337805));
#25645=CARTESIAN_POINT('Ctrl Pts',(65.1296671539667,93.5724251671486,207.285549615094));
#25646=CARTESIAN_POINT('Origin',(64.9174359473229,93.7042420150737,207.276481344607));
#25647=CARTESIAN_POINT('Origin',(87.370415498102,95.4011189555928,207.276481344607));
#25648=CARTESIAN_POINT('',(87.1804067618325,95.2389020358428,207.285548914041));
#25649=CARTESIAN_POINT('',(87.1576445151781,95.5323763699572,207.276481344607));
#25650=CARTESIAN_POINT('Origin',(87.370415498102,95.4011189555928,207.276481344607));
#25651=CARTESIAN_POINT('',(87.235703204888,95.2016981816169,207.344186240766));
#25652=CARTESIAN_POINT('Ctrl Pts',(87.1804056812849,95.2389029103722,207.285549099905));
#25653=CARTESIAN_POINT('Ctrl Pts',(87.1813645562961,95.2382603596069,207.294146996371));
#25654=CARTESIAN_POINT('Ctrl Pts',(87.1837422934887,95.2366672287293,207.302683426847));
#25655=CARTESIAN_POINT('Ctrl Pts',(87.1898436571226,95.2325743250902,207.315496320451));
#25656=CARTESIAN_POINT('Ctrl Pts',(87.1928794417903,95.2305371396332,207.320274409274));
#25657=CARTESIAN_POINT('Ctrl Pts',(87.1998212692631,95.2258745498999,207.328654585832));
#25658=CARTESIAN_POINT('Ctrl Pts',(87.2037283980161,95.2232484545878,207.332255389428));
#25659=CARTESIAN_POINT('Ctrl Pts',(87.211851391824,95.2177833855431,207.337933035602));
#25660=CARTESIAN_POINT('Ctrl Pts',(87.2164816625401,95.2146657032897,207.340322634924));
#25661=CARTESIAN_POINT('Ctrl Pts',(87.2261075175784,95.2081768430205,207.343449242348));
#25662=CARTESIAN_POINT('Ctrl Pts',(87.231103089383,95.2048056417694,207.344186240766));
#25663=CARTESIAN_POINT('Ctrl Pts',(87.235703204888,95.2016981816168,207.344186240766));
#25664=CARTESIAN_POINT('',(87.370415498102,95.4011189555928,207.526481344607));
#25665=CARTESIAN_POINT('Origin',(87.370415498102,95.4011189555928,207.276481344607));
#25666=CARTESIAN_POINT('Origin',(87.370415498102,95.4011189555928,207.276481344607));
#25667=CARTESIAN_POINT('Origin',(65.3426635064322,95.5210854135286,207.276481344607));
#25668=CARTESIAN_POINT('',(65.1884661129904,95.7178674346986,207.276481344607));
#25669=CARTESIAN_POINT('',(65.1520804375556,95.3592889554166,207.276481344607));
#25670=CARTESIAN_POINT('Origin',(65.3426635064322,95.5210854135286,207.276481344607));
#25671=CARTESIAN_POINT('',(65.3426635064322,95.5210854135286,207.526481344607));
#25672=CARTESIAN_POINT('Origin',(65.3426635064322,95.5210854135286,207.276481344607));
#25673=CARTESIAN_POINT('Origin',(65.3426635064322,95.5210854135286,207.276481344607));
#25674=CARTESIAN_POINT('Origin',(86.6766969576459,97.1335683214121,207.276481344607));
#25675=CARTESIAN_POINT('',(86.7995649337003,97.3512916790481,207.276481344607));
#25676=CARTESIAN_POINT('',(86.6766969576459,97.1335683214121,207.526481344607));
#25677=CARTESIAN_POINT('Origin',(86.6766969576459,97.1335683214121,207.276481344607));
#25678=CARTESIAN_POINT('',(86.8894679405697,97.0023109070477,207.276481344607));
#25679=CARTESIAN_POINT('Origin',(86.6766969576459,97.1335683214121,207.276481344607));
#25680=CARTESIAN_POINT('Origin',(86.6766969576459,97.1335683214121,207.276481344607));
#25681=CARTESIAN_POINT('Origin',(77.215862801455,80.368869783441,207.2));
#25682=CARTESIAN_POINT('',(82.4344268912437,95.2821721957428,207.2));
#25683=CARTESIAN_POINT('Origin',(77.215862801455,80.368869783441,207.2));
#25684=CARTESIAN_POINT('',(82.335340231311,94.999008225889,207.5));
#25685=CARTESIAN_POINT('Origin',(82.335340231311,94.999008225889,207.2));
#25686=CARTESIAN_POINT('Origin',(77.215862801455,80.368869783441,207.5));
#25687=CARTESIAN_POINT('Origin',(77.215862801455,80.368869783441,209.104699448314));
#25688=CARTESIAN_POINT('',(87.6199620943882,110.101086618093,209.104699448314));
#25689=CARTESIAN_POINT('',(66.8117635085218,50.6366529487886,209.104699448314));
#25690=CARTESIAN_POINT('Origin',(77.215862801455,80.368869783441,209.104699448314));
#25691=CARTESIAN_POINT('Origin',(77.215862801455,80.368869783441,209.104699448314));
#25692=CARTESIAN_POINT('',(66.9092858372326,50.9153464658161,209.404662059183));
#25693=CARTESIAN_POINT('Origin',(66.9108501684545,50.9198169186424,209.104699448314));
#25694=CARTESIAN_POINT('Origin',(77.215862801455,80.368869783441,209.404662059183));
#25695=CARTESIAN_POINT('Origin',(77.215862801455,80.368869783441,209.995300551686));
#25696=CARTESIAN_POINT('',(81.344473631984,92.1673685273507,209.995300551686));
#25697=CARTESIAN_POINT('Origin',(77.215862801455,80.368869783441,209.995300551686));
#25698=CARTESIAN_POINT('',(81.4419959606949,92.4460620443781,209.695337940817));
#25699=CARTESIAN_POINT('Origin',(81.4435602919167,92.4505324972045,209.995300551686));
#25700=CARTESIAN_POINT('',(72.9897296422151,68.2916775225039,209.695337940817));
#25701=CARTESIAN_POINT('Origin',(77.215862801455,80.368869783441,209.695337940817));
#25702=CARTESIAN_POINT('Origin',(77.215862801455,80.368869783441,209.695337940817));
#25703=CARTESIAN_POINT('Origin',(77.215862801455,80.368869783441,207.8));
#25704=CARTESIAN_POINT('',(80.6838958990994,90.2796087283251,207.5));
#25705=CARTESIAN_POINT('Origin',(77.215862801455,80.368869783441,207.5));
#25706=CARTESIAN_POINT('',(80.5848092391667,89.9964447584713,207.8));
#25707=CARTESIAN_POINT('Origin',(80.6838958990994,90.2796087283251,207.8));
#25708=CARTESIAN_POINT('Origin',(77.215862801455,80.368869783441,207.8));
#25709=CARTESIAN_POINT('Origin',(77.215862801455,80.368869783441,209.7));
#25710=CARTESIAN_POINT('',(73.7478297038106,70.4581308385569,210.));
#25711=CARTESIAN_POINT('Origin',(77.215862801455,80.368869783441,210.));
#25712=CARTESIAN_POINT('',(73.8469163637433,70.7412948084107,209.7));
#25713=CARTESIAN_POINT('Origin',(73.7478297038106,70.4581308385569,209.7));
#25714=CARTESIAN_POINT('',(80.5848092391667,89.9964447584713,209.7));
#25715=CARTESIAN_POINT('Origin',(77.215862801455,80.368869783441,209.7));
#25716=CARTESIAN_POINT('Origin',(77.215862801455,80.368869783441,209.7));
#25717=CARTESIAN_POINT('Origin',(77.215862801455,80.368869783441,208.4));
#25718=CARTESIAN_POINT('',(87.6199620943882,110.101086618093,208.4));
#25719=CARTESIAN_POINT('Origin',(77.215862801455,80.368869783441,208.4));
#25720=CARTESIAN_POINT('',(87.5208754344555,109.81792264824,208.1));
#25721=CARTESIAN_POINT('Origin',(87.5208754344555,109.81792264824,208.4));
#25722=CARTESIAN_POINT('Origin',(77.215862801455,80.368869783441,208.1));
#25723=CARTESIAN_POINT('Origin',(77.215862801455,80.368869783441,207.8));
#25724=CARTESIAN_POINT('',(83.2271201707053,97.5474839545735,208.1));
#25725=CARTESIAN_POINT('Origin',(77.215862801455,80.368869783441,208.1));
#25726=CARTESIAN_POINT('',(83.1280335107726,97.2643199847197,207.8));
#25727=CARTESIAN_POINT('Origin',(83.2271201707053,97.5474839545735,207.8));
#25728=CARTESIAN_POINT('Origin',(77.215862801455,80.368869783441,207.8));
#25729=CARTESIAN_POINT('Origin',(77.215862801455,80.368869783441,198.));
#25730=CARTESIAN_POINT('',(83.000126282037,96.8987943056185,197.986679815914));
#25731=CARTESIAN_POINT('Origin',(77.215862801455,80.368869783441,197.986679815914));
#25732=CARTESIAN_POINT('',(82.9011373407276,96.6159095902407,197.7));
#25733=CARTESIAN_POINT('Origin',(82.9011373407276,96.6159095902407,198.));
#25734=CARTESIAN_POINT('Origin',(77.215862801455,80.368869783441,197.7));
#25735=CARTESIAN_POINT('Origin',(77.215862801455,80.368869783441,198.));
#25736=CARTESIAN_POINT('',(82.5335135511764,95.5653361655966,197.7));
#25737=CARTESIAN_POINT('Origin',(77.215862801455,80.368869783441,197.7));
#25738=CARTESIAN_POINT('',(82.4344268912437,95.2821721957428,198.));
#25739=CARTESIAN_POINT('Origin',(82.5335135511764,95.5653361655966,198.));
#25740=CARTESIAN_POINT('Origin',(77.215862801455,80.368869783441,198.));
#25741=CARTESIAN_POINT('Origin',(77.215862801455,80.368869783441,209.7));
#25742=CARTESIAN_POINT('',(87.6199620943882,110.101086618093,209.7));
#25743=CARTESIAN_POINT('Origin',(77.215862801455,80.368869783441,209.7));
#25744=CARTESIAN_POINT('',(83.1280335107726,97.2643199847197,207.344186240766));
#25745=CARTESIAN_POINT('',(83.1280335107726,97.2643199847197,209.7));
#25746=CARTESIAN_POINT('',(66.2091808261905,94.4849227691515,207.344186240766));
#25747=CARTESIAN_POINT('Origin',(77.215862801455,80.368869783441,207.344186240766));
#25748=CARTESIAN_POINT('',(66.156698979235,94.4438437095257,207.285548215601));
#25749=CARTESIAN_POINT('Ctrl Pts',(66.156697797991,94.4438429424263,207.285548403906));
#25750=CARTESIAN_POINT('Ctrl Pts',(66.157605358421,94.4445560422264,207.294146535105));
#25751=CARTESIAN_POINT('Ctrl Pts',(66.1598557893509,94.4463245033558,207.302683220627));
#25752=CARTESIAN_POINT('Ctrl Pts',(66.1656351357801,94.4508609547001,207.315496320451));
#25753=CARTESIAN_POINT('Ctrl Pts',(66.1685113430769,94.4531178429828,207.320274409274));
#25754=CARTESIAN_POINT('Ctrl Pts',(66.1750922888656,94.4582772871593,207.328654585832));
#25755=CARTESIAN_POINT('Ctrl Pts',(66.1787980203727,94.4611806620366,207.332255389429));
#25756=CARTESIAN_POINT('Ctrl Pts',(66.1865074101033,94.4672151726256,207.337933035602));
#25757=CARTESIAN_POINT('Ctrl Pts',(66.1909042788197,94.4706541979277,207.340322634924));
#25758=CARTESIAN_POINT('Ctrl Pts',(66.2000520670299,94.4778012507239,207.343449242348));
#25759=CARTESIAN_POINT('Ctrl Pts',(66.2048030047484,94.4815092591281,207.344186240766));
#25760=CARTESIAN_POINT('Ctrl Pts',(66.2091808261905,94.4849227691515,207.344186240766));
#25761=CARTESIAN_POINT('',(66.1149823135236,94.4109655092461,206.699999966761));
#25762=CARTESIAN_POINT('Ctrl Pts',(66.114982666556,94.4109657890452,206.69999993673));
#25763=CARTESIAN_POINT('Ctrl Pts',(66.1225753392106,94.4169681229566,206.845179687536));
#25764=CARTESIAN_POINT('Ctrl Pts',(66.1311276201516,94.4237204506714,206.987155428366));
#25765=CARTESIAN_POINT('Ctrl Pts',(66.1458107299093,94.4352827739518,207.172140952524));
#25766=CARTESIAN_POINT('Ctrl Pts',(66.1507290952786,94.4391531397854,207.228982204513));
#25767=CARTESIAN_POINT('Ctrl Pts',(66.1567000620981,94.4438447214087,207.285548017371));
#25768=CARTESIAN_POINT('',(65.1689064613399,93.6082369448483,206.699999825671));
#25769=CARTESIAN_POINT('Origin',(77.215862801455,80.368869783441,206.7));
#25770=CARTESIAN_POINT('Ctrl Pts',(65.1296586956086,93.5724174245798,207.285548075353));
#25771=CARTESIAN_POINT('Ctrl Pts',(65.1353053901753,93.5775862704772,207.228541407465));
#25772=CARTESIAN_POINT('Ctrl Pts',(65.1399579139802,93.5818387450385,207.17122564234));
#25773=CARTESIAN_POINT('Ctrl Pts',(65.153736689073,93.5944243404895,206.986234752513));
#25774=CARTESIAN_POINT('Ctrl Pts',(65.1617661917048,93.6017397697266,206.84471856995));
#25775=CARTESIAN_POINT('Ctrl Pts',(65.1689047120699,93.6082353570854,206.699999668119));
#25776=CARTESIAN_POINT('Origin',(77.215862801455,80.368869783441,207.344186240766));
#25777=CARTESIAN_POINT('',(60.4296192316701,74.1534030434687,206.699999966494));
#25778=CARTESIAN_POINT('Ctrl Pts',(60.4296190734685,74.1534034691059,206.699999936224));
#25779=CARTESIAN_POINT('Ctrl Pts',(60.4262555077399,74.162487523505,206.845315153431));
#25780=CARTESIAN_POINT('Ctrl Pts',(60.4224746505866,74.1727180566403,206.987426060047));
#25781=CARTESIAN_POINT('Ctrl Pts',(60.4160156054915,74.1902646513169,207.172409754229));
#25782=CARTESIAN_POINT('Ctrl Pts',(60.4138599947734,74.1961265458095,207.229111613155));
#25783=CARTESIAN_POINT('Ctrl Pts',(60.4112505043822,74.2032387901793,207.285547584101));
#25784=CARTESIAN_POINT('',(60.9005109638373,73.0054945851509,206.699999827092));
#25785=CARTESIAN_POINT('Origin',(77.215862801455,80.368869783441,206.7));
#25786=CARTESIAN_POINT('',(60.9224377356629,72.9571021383096,207.285550046838));
#25787=CARTESIAN_POINT('Ctrl Pts',(60.9224424447625,72.957091786218,207.285548519515));
#25788=CARTESIAN_POINT('Ctrl Pts',(60.9192653221022,72.964076101594,207.228412061246));
#25789=CARTESIAN_POINT('Ctrl Pts',(60.9166543398919,72.969827192782,207.170956688005));
#25790=CARTESIAN_POINT('Ctrl Pts',(60.9089490604414,72.9868142803523,206.985964005474));
#25791=CARTESIAN_POINT('Ctrl Pts',(60.904478835706,72.9967027942644,206.844583002872));
#25792=CARTESIAN_POINT('Ctrl Pts',(60.9005119250647,73.0054924482591,206.699999670811));
#25793=CARTESIAN_POINT('',(60.95014735807,72.8964872239874,207.344186240766));
#25794=CARTESIAN_POINT('Ctrl Pts',(60.95014735807,72.8964872239874,207.344186240766));
#25795=CARTESIAN_POINT('Ctrl Pts',(60.9478299428105,72.9015317217597,207.344186240766));
#25796=CARTESIAN_POINT('Ctrl Pts',(60.9453166586466,72.9070093250897,207.343449242348));
#25797=CARTESIAN_POINT('Ctrl Pts',(60.9404808057933,72.9175628515142,207.340322634924));
#25798=CARTESIAN_POINT('Ctrl Pts',(60.9381582121413,72.9226387660393,207.337933035602));
#25799=CARTESIAN_POINT('Ctrl Pts',(60.9340879278448,72.9315428546402,207.332255389429));
#25800=CARTESIAN_POINT('Ctrl Pts',(60.932132684209,72.9358252668116,207.328654585832));
#25801=CARTESIAN_POINT('Ctrl Pts',(60.9286619592505,72.9434333401516,207.320274409274));
#25802=CARTESIAN_POINT('Ctrl Pts',(60.9271459728306,72.9467601852501,207.315496320451));
#25803=CARTESIAN_POINT('Ctrl Pts',(60.9241006297042,72.9534461421773,207.302683707375));
#25804=CARTESIAN_POINT('Ctrl Pts',(60.922915707046,72.9560514050313,207.294147623841));
#25805=CARTESIAN_POINT('Ctrl Pts',(60.9224377356548,72.9571021383274,207.285550046692));
#25806=CARTESIAN_POINT('',(77.8232478055421,62.47917768277,207.344186240766));
#25807=CARTESIAN_POINT('Origin',(77.215862801455,80.368869783441,207.344186240766));
#25808=CARTESIAN_POINT('',(77.889852177038,62.4815632844674,207.285548215602));
#25809=CARTESIAN_POINT('Ctrl Pts',(77.8898535835874,62.4815632107454,207.285548403908));
#25810=CARTESIAN_POINT('Ctrl Pts',(77.88870020223,62.4815197515247,207.294146535107));
#25811=CARTESIAN_POINT('Ctrl Pts',(77.885840089992,62.481411806529,207.302683220628));
#25812=CARTESIAN_POINT('Ctrl Pts',(77.8784980413168,62.4811387548963,207.315496320451));
#25813=CARTESIAN_POINT('Ctrl Pts',(77.8748445750857,62.4810034861528,207.320274409275));
#25814=CARTESIAN_POINT('Ctrl Pts',(77.8664878329066,62.4806975910132,207.328654585832));
#25815=CARTESIAN_POINT('Ctrl Pts',(77.861783272206,62.4805268857253,207.332255389429));
#25816=CARTESIAN_POINT('Ctrl Pts',(77.8519992485687,62.4801763296939,207.337933035602));
#25817=CARTESIAN_POINT('Ctrl Pts',(77.8464206987003,62.4799785143681,207.340322634924));
#25818=CARTESIAN_POINT('Ctrl Pts',(77.8348190503462,62.4795733621974,207.343449242348));
#25819=CARTESIAN_POINT('Ctrl Pts',(77.8287959483374,62.4793660515086,207.344186240766));
#25820=CARTESIAN_POINT('Ctrl Pts',(77.8232478055421,62.47917768277,207.344186240766));
#25821=CARTESIAN_POINT('',(77.9429269897965,62.483641866357,206.699999966761));
#25822=CARTESIAN_POINT('Ctrl Pts',(77.9429265397247,62.483641847502,206.699999936729));
#25823=CARTESIAN_POINT('Ctrl Pts',(77.9332558551646,62.4832487183737,206.845179687469));
#25824=CARTESIAN_POINT('Ctrl Pts',(77.9223679958966,62.4828128751116,206.987155428232));
#25825=CARTESIAN_POINT('Ctrl Pts',(77.9036929474648,62.4820892744566,207.172140952389));
#25826=CARTESIAN_POINT('Ctrl Pts',(77.89743896233,62.4818490253519,207.228982204448));
#25827=CARTESIAN_POINT('Ctrl Pts',(77.8898507061996,62.4815631023261,207.285548017369));
#25828=CARTESIAN_POINT('',(79.1801504439358,62.5769734833615,206.699999825671));
#25829=CARTESIAN_POINT('Origin',(77.215862801455,80.368869783441,206.7));
#25830=CARTESIAN_POINT('Ctrl Pts',(79.2329567391591,62.5828828261064,207.285548075332));
#25831=CARTESIAN_POINT('Ctrl Pts',(79.225350295901,62.5820201857243,207.228541407435));
#25832=CARTESIAN_POINT('Ctrl Pts',(79.219086783242,62.5813145464144,207.171225642298));
#25833=CARTESIAN_POINT('Ctrl Pts',(79.200541892634,62.5792315466046,206.986234752478));
#25834=CARTESIAN_POINT('Ctrl Pts',(79.1897459871301,62.5780328632611,206.844718569932));
#25835=CARTESIAN_POINT('Ctrl Pts',(79.1801527923866,62.5769737396933,206.69999966812));
#25836=CARTESIAN_POINT('',(94.419021870213,75.4230313252008,207.344186240766));
#25837=CARTESIAN_POINT('Origin',(77.215862801455,80.368869783441,207.344186240766));
#25838=CARTESIAN_POINT('',(94.4373172975837,75.4871179909361,207.285548914041));
#25839=CARTESIAN_POINT('Ctrl Pts',(94.4373177953928,75.4871192888155,207.285549099901));
#25840=CARTESIAN_POINT('Ctrl Pts',(94.4370030019744,75.4860087853819,207.294146996368));
#25841=CARTESIAN_POINT('Ctrl Pts',(94.4362226056726,75.4832551184153,207.302683426846));
#25842=CARTESIAN_POINT('Ctrl Pts',(94.4342154480476,75.4761875999915,207.315496320451));
#25843=CARTESIAN_POINT('Ctrl Pts',(94.4332160785974,75.4726708722743,207.320274409274));
#25844=CARTESIAN_POINT('Ctrl Pts',(94.4309268349098,75.4646279825559,207.328654585832));
#25845=CARTESIAN_POINT('Ctrl Pts',(94.4296366390347,75.4601005742151,207.332255389429));
#25846=CARTESIAN_POINT('Ctrl Pts',(94.4269491926396,75.4506863488119,207.337933035602));
#25847=CARTESIAN_POINT('Ctrl Pts',(94.4254149329567,75.4453192828758,207.340322634924));
#25848=CARTESIAN_POINT('Ctrl Pts',(94.4222182129065,75.4341593826194,207.343449242348));
#25849=CARTESIAN_POINT('Ctrl Pts',(94.4205557265731,75.428366553024,207.344186240766));
#25850=CARTESIAN_POINT('Ctrl Pts',(94.419021870213,75.4230313252008,207.344186240766));
#25851=CARTESIAN_POINT('',(94.4517290859501,75.5382473180358,206.699999967191));
#25852=CARTESIAN_POINT('Ctrl Pts',(94.4517289664912,75.5382468897594,206.699999937545));
#25853=CARTESIAN_POINT('Ctrl Pts',(94.4491205523975,75.528939958291,206.844960355996));
#25854=CARTESIAN_POINT('Ctrl Pts',(94.44617790075,75.5184654593862,206.986717295167));
#25855=CARTESIAN_POINT('Ctrl Pts',(94.44110395422,75.5004927769422,207.171705759969));
#25856=CARTESIAN_POINT('Ctrl Pts',(94.4393958410628,75.4944500502634,207.228772753636));
#25857=CARTESIAN_POINT('Ctrl Pts',(94.4373170203668,75.4871165547408,207.285548718384));
#25858=CARTESIAN_POINT('',(94.7449571171753,76.7438384229745,206.69999982336));
#25859=CARTESIAN_POINT('Origin',(77.215862801455,80.368869783441,206.7));
#25860=CARTESIAN_POINT('',(94.7556372114542,76.7958719320097,207.285548916829));
#25861=CARTESIAN_POINT('Ctrl Pts',(94.7556395308917,76.7958833180998,207.28554735655));
#25862=CARTESIAN_POINT('Ctrl Pts',(94.7541172320878,76.7884103591634,207.228750629597));
#25863=CARTESIAN_POINT('Ctrl Pts',(94.7528586977031,76.7822554461689,207.171660554524));
#25864=CARTESIAN_POINT('Ctrl Pts',(94.7491113652146,76.7639598982199,206.9866725855));
#25865=CARTESIAN_POINT('Ctrl Pts',(94.7469148396517,76.7533051195487,206.844937777645));
#25866=CARTESIAN_POINT('Ctrl Pts',(94.7449576048465,76.7438407664931,206.699999663745));
#25867=CARTESIAN_POINT('',(94.7688192182643,76.861203746089,207.344186240769));
#25868=CARTESIAN_POINT('Ctrl Pts',(94.7688192182643,76.861203746089,207.344186240766));
#25869=CARTESIAN_POINT('Ctrl Pts',(94.7677313833287,76.8557600353682,207.344186240766));
#25870=CARTESIAN_POINT('Ctrl Pts',(94.766547643411,76.8498507633878,207.343449242348));
#25871=CARTESIAN_POINT('Ctrl Pts',(94.7642617790702,76.8384693216063,207.340322634924));
#25872=CARTESIAN_POINT('Ctrl Pts',(94.7631596798826,76.8329971440765,207.337933035602));
#25873=CARTESIAN_POINT('Ctrl Pts',(94.7612231800783,76.8234002708056,207.332255389429));
#25874=CARTESIAN_POINT('Ctrl Pts',(94.7602899163563,76.8187860481728,207.328654585832));
#25875=CARTESIAN_POINT('Ctrl Pts',(94.7586295191669,76.8105902082001,207.320274409275));
#25876=CARTESIAN_POINT('Ctrl Pts',(94.7579020989926,76.8070073360248,207.315496320451));
#25877=CARTESIAN_POINT('Ctrl Pts',(94.7564390863843,76.7998074367317,207.302683372569));
#25878=CARTESIAN_POINT('Ctrl Pts',(94.7558676085502,76.7970029467077,207.294146874964));
#25879=CARTESIAN_POINT('Ctrl Pts',(94.7556372114512,76.7958719319941,207.285548916715));
#25880=CARTESIAN_POINT('Origin',(77.215862801455,80.368869783441,207.344186240766));
#25881=CARTESIAN_POINT('',(87.1362333696184,95.2684082920857,206.699999967189));
#25882=CARTESIAN_POINT('Ctrl Pts',(87.1362337400429,95.2684080461128,206.699999937541));
#25883=CARTESIAN_POINT('Ctrl Pts',(87.1442791135725,95.2630512969072,206.844960355813));
#25884=CARTESIAN_POINT('Ctrl Pts',(87.1533316246345,95.2570158707191,206.986717294808));
#25885=CARTESIAN_POINT('Ctrl Pts',(87.1688567256818,95.2466363964988,207.171705759608));
#25886=CARTESIAN_POINT('Ctrl Pts',(87.1740758642901,95.2431445791019,207.228772753463));
#25887=CARTESIAN_POINT('Ctrl Pts',(87.180408042097,95.2389013283705,207.28554871838));
#25888=CARTESIAN_POINT('',(86.0802605381687,95.9198328616278,206.699999823361));
#25889=CARTESIAN_POINT('Origin',(77.215862801455,80.368869783441,206.7));
#25890=CARTESIAN_POINT('',(86.0342766273764,95.946016145882,207.285410051862));
#25891=CARTESIAN_POINT('Ctrl Pts',(86.0340971970359,95.9460563761667,207.285262733977));
#25892=CARTESIAN_POINT('Ctrl Pts',(86.0407188285758,95.9423078752001,207.228559905421));
#25893=CARTESIAN_POINT('Ctrl Pts',(86.0461731162624,95.9392149023471,207.171573816788));
#25894=CARTESIAN_POINT('Ctrl Pts',(86.0624076112581,95.9300016641009,206.986672585795));
#25895=CARTESIAN_POINT('Ctrl Pts',(86.0718621442226,95.9246201364663,206.844937777794));
#25896=CARTESIAN_POINT('Ctrl Pts',(86.0802584600576,95.9198340496126,206.699999663746));
#25897=CARTESIAN_POINT('',(85.9760132775813,95.9787949477595,207.34418624088));
#25898=CARTESIAN_POINT('Ctrl Pts',(85.9760132775813,95.9787949477595,207.344186240766));
#25899=CARTESIAN_POINT('Ctrl Pts',(85.980854394653,95.9760781561302,207.344186240766));
#25900=CARTESIAN_POINT('Ctrl Pts',(85.9861086505249,95.9731262871016,207.343449242348));
#25901=CARTESIAN_POINT('Ctrl Pts',(85.9962266739679,95.9674352419939,207.340322634924));
#25902=CARTESIAN_POINT('Ctrl Pts',(86.0010904566875,95.9646960875269,207.337933035602));
#25903=CARTESIAN_POINT('Ctrl Pts',(86.0096192141986,95.9598887698357,207.332255389428));
#25904=CARTESIAN_POINT('Ctrl Pts',(86.0137192063509,95.9575753100821,207.328654585832));
#25905=CARTESIAN_POINT('Ctrl Pts',(86.0210008224145,95.9534635246808,207.320274409274));
#25906=CARTESIAN_POINT('Ctrl Pts',(86.024183551148,95.9516645385931,207.315496320451));
#25907=CARTESIAN_POINT('Ctrl Pts',(86.0306209260497,95.9480245135938,207.302599308419));
#25908=CARTESIAN_POINT('Ctrl Pts',(86.0331233851216,95.9466076511945,207.293958732845));
#25909=CARTESIAN_POINT('Ctrl Pts',(86.0341066806811,95.946051007478,207.285265181889));
#25910=CARTESIAN_POINT('Origin',(77.215862801455,80.368869783441,207.344186240766));
#25911=CARTESIAN_POINT('Origin',(77.215862801455,80.368869783441,197.7));
#25912=CARTESIAN_POINT('',(77.807098035462,62.6991535162084,201.741111932487));
#25913=CARTESIAN_POINT('',(61.1539813020695,72.980744529632,201.741111932425));
#25914=CARTESIAN_POINT('Origin',(77.215862801455,80.368869783441,201.741111932358));
#25915=CARTESIAN_POINT('Ctrl Pts',(60.9005100041822,73.0054967262931,206.699999797758));
#25916=CARTESIAN_POINT('Ctrl Pts',(60.9383106449015,73.0111068965595,205.87285383463));
#25917=CARTESIAN_POINT('Ctrl Pts',(60.9765983511668,73.0156536991714,205.045723649382));
#25918=CARTESIAN_POINT('Ctrl Pts',(61.036177641715,73.017794419973,203.805110977245));
#25919=CARTESIAN_POINT('Ctrl Pts',(61.056362889984,73.0177980538245,203.391593008183));
#25920=CARTESIAN_POINT('Ctrl Pts',(61.0881220477898,73.0145739609718,202.771407903025));
#25921=CARTESIAN_POINT('Ctrl Pts',(61.0989324419101,73.0130108881507,202.564693369105));
#25922=CARTESIAN_POINT('Ctrl Pts',(61.1161852013738,73.0084051153063,202.254685622264));
#25923=CARTESIAN_POINT('Ctrl Pts',(61.1220930802366,73.0065284737844,202.151351857905));
#25924=CARTESIAN_POINT('Ctrl Pts',(61.1316846267869,73.0021175223093,201.996443305138));
#25925=CARTESIAN_POINT('Ctrl Pts',(61.1349921347903,73.0004066620236,201.944814005535));
#25926=CARTESIAN_POINT('Ctrl Pts',(61.1404702932454,72.9967068289114,201.86746331438));
#25927=CARTESIAN_POINT('Ctrl Pts',(61.1423745128547,72.9953029618212,201.841686059695));
#25928=CARTESIAN_POINT('Ctrl Pts',(61.1455990957178,72.9923866534762,201.803113993957));
#25929=CARTESIAN_POINT('Ctrl Pts',(61.1467287621209,72.9912937104118,201.790272644151));
#25930=CARTESIAN_POINT('Ctrl Pts',(61.1486890600559,72.9890682219378,201.771088244947));
#25931=CARTESIAN_POINT('Ctrl Pts',(61.1493825770163,72.9882385880473,201.764699691419));
#25932=CARTESIAN_POINT('Ctrl Pts',(61.1506142386167,72.9865676498396,201.755215001631));
#25933=CARTESIAN_POINT('Ctrl Pts',(61.1510536238296,72.9859469806554,201.752062963043));
#25934=CARTESIAN_POINT('Ctrl Pts',(61.1521195445798,72.9842847677176,201.745890878911));
#25935=CARTESIAN_POINT('Ctrl Pts',(61.1526220601575,72.9836995364303,201.741111962039));
#25936=CARTESIAN_POINT('Ctrl Pts',(61.1539813021289,72.9807445296591,201.741111932358));
#25937=CARTESIAN_POINT('',(60.5926319978065,74.3491829381161,201.741111932489));
#25938=CARTESIAN_POINT('Ctrl Pts',(60.5926319978361,74.3491829381273,201.741111932358));
#25939=CARTESIAN_POINT('Ctrl Pts',(60.5937393175791,74.3461250955133,201.741111963319));
#25940=CARTESIAN_POINT('Ctrl Pts',(60.5937927553975,74.3453549761292,201.745890861414));
#25941=CARTESIAN_POINT('Ctrl Pts',(60.5942012600518,74.3434228683981,201.752062897732));
#25942=CARTESIAN_POINT('Ctrl Pts',(60.594324352301,74.3426723409001,201.75521490968));
#25943=CARTESIAN_POINT('Ctrl Pts',(60.5946210288793,74.3406175201717,201.764699543009));
#25944=CARTESIAN_POINT('Ctrl Pts',(60.5947099819196,74.3395396558076,201.771088063263));
#25945=CARTESIAN_POINT('Ctrl Pts',(60.5948774701612,74.3365780380361,201.790272386922));
#25946=CARTESIAN_POINT('Ctrl Pts',(60.5948409011576,74.3350062230635,201.80311369854));
#25947=CARTESIAN_POINT('Ctrl Pts',(60.5945936658665,74.3306643267586,201.841685661127));
#25948=CARTESIAN_POINT('Ctrl Pts',(60.5942241686695,74.3283268124689,201.867462868231));
#25949=CARTESIAN_POINT('Ctrl Pts',(60.5929232339402,74.3218432894536,201.944813434034));
#25950=CARTESIAN_POINT('Ctrl Pts',(60.5917705844262,74.3183009330135,201.996442677713));
#25951=CARTESIAN_POINT('Ctrl Pts',(60.5880415026138,74.3084200407889,202.151351090415));
#25952=CARTESIAN_POINT('Ctrl Pts',(60.5851546003288,74.3029318988099,202.254684800762));
#25953=CARTESIAN_POINT('Ctrl Pts',(60.5761099141485,74.2875272696542,202.56469242477));
#25954=CARTESIAN_POINT('Ctrl Pts',(60.5695137820587,74.2788162752227,202.771406933039));
#25955=CARTESIAN_POINT('Ctrl Pts',(60.5491749431726,74.2541982851575,203.391592016162));
#25956=CARTESIAN_POINT('Ctrl Pts',(60.5348068091768,74.2400125818057,203.805110051126));
#25957=CARTESIAN_POINT('Ctrl Pts',(60.490901938456,74.1996574574576,205.045723068922));
#25958=CARTESIAN_POINT('Ctrl Pts',(60.4604606428822,74.1759805013104,205.872853625126));
#25959=CARTESIAN_POINT('Ctrl Pts',(60.4296193906672,74.1534026174594,206.699999960794));
#25960=CARTESIAN_POINT('',(65.2237133691081,93.3595119561188,201.741111932425));
#25961=CARTESIAN_POINT('Origin',(77.215862801455,80.368869783441,201.741111932358));
#25962=CARTESIAN_POINT('Ctrl Pts',(65.1689082151754,93.6082385324285,206.69999979608));
#25963=CARTESIAN_POINT('Ctrl Pts',(65.1859267393918,93.5740209471359,205.872853767758));
#25964=CARTESIAN_POINT('Ctrl Pts',(65.202084596116,93.5390113872842,205.045723525105));
#25965=CARTESIAN_POINT('Ctrl Pts',(65.2225352272511,93.483007739342,203.805110800395));
#25966=CARTESIAN_POINT('Ctrl Pts',(65.2287775850782,93.4638108194459,203.391592818749));
#25967=CARTESIAN_POINT('Ctrl Pts',(65.2355278034753,93.4326082192978,202.771407717802));
#25968=CARTESIAN_POINT('Ctrl Pts',(65.2373826894445,93.4218433237596,202.564693188781));
#25969=CARTESIAN_POINT('Ctrl Pts',(65.2383353173637,93.4040105223618,202.2546854654));
#25970=CARTESIAN_POINT('Ctrl Pts',(65.2383767315617,93.3978114373734,202.151351711356));
#25971=CARTESIAN_POINT('Ctrl Pts',(65.2371466798792,93.3873253878303,201.996443185339));
#25972=CARTESIAN_POINT('Ctrl Pts',(65.2365420159416,93.3836507465764,201.944813896416));
#25973=CARTESIAN_POINT('Ctrl Pts',(65.2347168317198,93.3772967459819,201.8674632292));
#25974=CARTESIAN_POINT('Ctrl Pts',(65.233970373536,93.3750516660578,201.841685983602));
#25975=CARTESIAN_POINT('Ctrl Pts',(65.2321937479147,93.3710832436713,201.803113937563));
#25976=CARTESIAN_POINT('Ctrl Pts',(65.2315035646884,93.369670954703,201.79027259505));
#25977=CARTESIAN_POINT('Ctrl Pts',(65.2299931117319,93.3671185443332,201.771088210274));
#25978=CARTESIAN_POINT('Ctrl Pts',(65.2294185185355,93.3662024733727,201.764699663099));
#25979=CARTESIAN_POINT('Ctrl Pts',(65.2282102113793,93.3645144973317,201.755214984094));
#25980=CARTESIAN_POINT('Ctrl Pts',(65.2277557874688,93.3639047286458,201.752062950593));
#25981=CARTESIAN_POINT('Ctrl Pts',(65.2265045506743,93.3623770854172,201.745890875594));
#25982=CARTESIAN_POINT('Ctrl Pts',(65.2261032722959,93.3617181671861,201.741111962317));
#25983=CARTESIAN_POINT('Ctrl Pts',(65.2237133691526,93.3595119560702,201.741111932358));
#25984=CARTESIAN_POINT('',(66.3515448153964,94.3164511782291,201.741111932487));
#25985=CARTESIAN_POINT('Ctrl Pts',(66.3515448154396,94.3164511781742,201.741111932358));
#25986=CARTESIAN_POINT('Ctrl Pts',(66.3489790895714,94.3144526354332,201.741111963088));
#25987=CARTESIAN_POINT('Ctrl Pts',(66.3482633166899,94.314163781558,201.745890864771));
#25988=CARTESIAN_POINT('Ctrl Pts',(66.3465522068942,94.3131779463266,201.752062910219));
#25989=CARTESIAN_POINT('Ctrl Pts',(66.3458765257224,94.3128288491502,201.755214927256));
#25990=CARTESIAN_POINT('Ctrl Pts',(66.3440141578885,94.3119114361031,201.764699571368));
#25991=CARTESIAN_POINT('Ctrl Pts',(66.3430166397612,94.3114936124396,201.771088097978));
#25992=CARTESIAN_POINT('Ctrl Pts',(66.3402520120046,94.310418733184,201.790272436065));
#25993=CARTESIAN_POINT('Ctrl Pts',(66.3387459692438,94.3099675874997,201.803113754976));
#25994=CARTESIAN_POINT('Ctrl Pts',(66.3345405662682,94.308860434356,201.841685737264));
#25995=CARTESIAN_POINT('Ctrl Pts',(66.332203471895,94.3084892170732,201.867462953456));
#25996=CARTESIAN_POINT('Ctrl Pts',(66.3256357889722,94.3077221418656,201.9448135432));
#25997=CARTESIAN_POINT('Ctrl Pts',(66.3219108818743,94.3077232949242,201.99644279756));
#25998=CARTESIAN_POINT('Ctrl Pts',(66.3113619485989,94.3082153062037,202.151351237013));
#25999=CARTESIAN_POINT('Ctrl Pts',(66.3052506589714,94.3092643477764,202.254684957675));
#26000=CARTESIAN_POINT('Ctrl Pts',(66.2878059414537,94.3131043070356,202.564692605142));
#26001=CARTESIAN_POINT('Ctrl Pts',(66.2774834127232,94.3166848106869,202.77140711831));
#26002=CARTESIAN_POINT('Ctrl Pts',(66.247786403833,94.3284182028902,203.39159220564));
#26003=CARTESIAN_POINT('Ctrl Pts',(66.2298555084119,94.3376980668689,203.805110228017));
#26004=CARTESIAN_POINT('Ctrl Pts',(66.1779094279662,94.3669797255545,205.045723192665));
#26005=CARTESIAN_POINT('Ctrl Pts',(66.1459849127475,94.3886123873169,205.872853690893));
#26006=CARTESIAN_POINT('Ctrl Pts',(66.1149819603839,94.4109652285824,206.699999961109));
#26007=CARTESIAN_POINT('',(81.3941453425875,97.5476470120627,201.741111932492));
#26008=CARTESIAN_POINT('Origin',(77.215862801455,80.368869783441,201.741111932358));
#26009=CARTESIAN_POINT('',(83.0552394877203,97.0562935504538,201.741111932358));
#26010=CARTESIAN_POINT('Origin',(77.215862801455,80.368869783441,201.741111932358));
#26011=CARTESIAN_POINT('',(82.9959179641957,96.8867680249146,197.7));
#26012=CARTESIAN_POINT('',(85.8606360184079,95.7908128547202,201.741111932426));
#26013=CARTESIAN_POINT('Origin',(77.215862801455,80.368869783441,201.741111932358));
#26014=CARTESIAN_POINT('Ctrl Pts',(86.0802626175339,95.9198316691863,206.699999793354));
#26015=CARTESIAN_POINT('Ctrl Pts',(86.0529786776688,95.893069019184,205.872853659539));
#26016=CARTESIAN_POINT('Ctrl Pts',(86.0246754069566,95.8668798833011,205.045723323998));
#26017=CARTESIAN_POINT('Ctrl Pts',(85.9777312853402,95.8301174987039,203.805110514213));
#26018=CARTESIAN_POINT('Ctrl Pts',(85.961402457991,95.8182460959664,203.391592512203));
#26019=CARTESIAN_POINT('Ctrl Pts',(85.9338117707789,95.8021796651052,202.771407418065));
#26020=CARTESIAN_POINT('Ctrl Pts',(85.9241464704097,95.7970874106423,202.56469289697));
#26021=CARTESIAN_POINT('Ctrl Pts',(85.9074798068452,95.7906677381534,202.254685211545));
#26022=CARTESIAN_POINT('Ctrl Pts',(85.901596526642,95.788711626652,202.151351474192));
#26023=CARTESIAN_POINT('Ctrl Pts',(85.8912427589881,95.7866390298392,201.996442991456));
#26024=CARTESIAN_POINT('Ctrl Pts',(85.8875608017384,95.7860778159899,201.944813719815));
#26025=CARTESIAN_POINT('Ctrl Pts',(85.880953134623,95.785848738158,201.867463091334));
#26026=CARTESIAN_POINT('Ctrl Pts',(85.8785870294705,95.7858643697771,201.841685860439));
#26027=CARTESIAN_POINT('Ctrl Pts',(85.8742633490481,95.7863267288807,201.803113846275));
#26028=CARTESIAN_POINT('Ctrl Pts',(85.8727067264141,95.7865463446168,201.790272515562));
#26029=CARTESIAN_POINT('Ctrl Pts',(85.8698121308553,95.787193427246,201.771088154131));
#26030=CARTESIAN_POINT('Ctrl Pts',(85.8687632059339,95.7874565578042,201.764699617238));
#26031=CARTESIAN_POINT('Ctrl Pts',(85.8667841989931,95.7880836116175,201.75521495568));
#26032=CARTESIAN_POINT('Ctrl Pts',(85.8660637545444,95.7883271813326,201.75206293041));
#26033=CARTESIAN_POINT('Ctrl Pts',(85.8642239733752,95.7890446301688,201.745890870187));
#26034=CARTESIAN_POINT('Ctrl Pts',(85.8634730846983,95.7892225381229,201.741111962688));
#26035=CARTESIAN_POINT('Ctrl Pts',(85.8606360183751,95.7908128546621,201.741111932358));
#26036=CARTESIAN_POINT('',(87.1194741084993,95.014241582934,201.741111932485));
#26037=CARTESIAN_POINT('Ctrl Pts',(87.119474108461,95.0142415828767,201.741111932358));
#26038=CARTESIAN_POINT('Ctrl Pts',(87.1167799038052,95.0160634812828,201.741111962705));
#26039=CARTESIAN_POINT('Ctrl Pts',(87.1162839950345,95.0166547167802,201.745890870188));
#26040=CARTESIAN_POINT('Ctrl Pts',(87.1148173319683,95.0179769977751,201.752062930411));
#26041=CARTESIAN_POINT('Ctrl Pts',(87.1142764019131,95.0185115640335,201.755214955681));
#26042=CARTESIAN_POINT('Ctrl Pts',(87.112828054955,95.0199988286518,201.76469961724));
#26043=CARTESIAN_POINT('Ctrl Pts',(87.1121222584439,95.0208181774568,201.771088154132));
#26044=CARTESIAN_POINT('Ctrl Pts',(87.1102451985936,95.0231147065111,201.790272515564));
#26045=CARTESIAN_POINT('Ctrl Pts',(87.1093504930545,95.0244073035463,201.803113846276));
#26046=CARTESIAN_POINT('Ctrl Pts',(87.1069973056896,95.0280638726432,201.84168586044));
#26047=CARTESIAN_POINT('Ctrl Pts',(87.1059216935689,95.0301714201536,201.867463091335));
#26048=CARTESIAN_POINT('Ctrl Pts',(87.1031616387417,95.0361794014043,201.944813719816));
#26049=CARTESIAN_POINT('Ctrl Pts',(87.1020111401724,95.0397217344228,201.996442991457));
#26050=CARTESIAN_POINT('Ctrl Pts',(87.0992177879608,95.0499047273817,202.151351474193));
#26051=CARTESIAN_POINT('Ctrl Pts',(87.0983261869635,95.0560402310952,202.254685211547));
#26052=CARTESIAN_POINT('Ctrl Pts',(87.0965852479142,95.0738154666901,202.564692896971));
#26053=CARTESIAN_POINT('Ctrl Pts',(87.0967994361659,95.0847380675769,202.771407418066));
#26054=CARTESIAN_POINT('Ctrl Pts',(87.0987782199621,95.1166043606802,203.391592512204));
#26055=CARTESIAN_POINT('Ctrl Pts',(87.1020610131019,95.1365238003,203.805110514214));
#26056=CARTESIAN_POINT('Ctrl Pts',(87.1138518873724,95.1949720607912,205.045723392875));
#26057=CARTESIAN_POINT('Ctrl Pts',(87.1245574910124,95.2320171179916,205.872853797301));
#26058=CARTESIAN_POINT('Ctrl Pts',(87.1362329983495,95.2684085378955,206.699999961615));
#26059=CARTESIAN_POINT('',(94.5543840898835,76.9128443788708,201.741111932426));
#26060=CARTESIAN_POINT('Origin',(77.215862801455,80.368869783441,201.741111932358));
#26061=CARTESIAN_POINT('Ctrl Pts',(94.7449566256531,76.7438360768859,206.699999793353));
#26062=CARTESIAN_POINT('Ctrl Pts',(94.7110726318838,76.7615145320216,205.87285365954));
#26063=CARTESIAN_POINT('Ctrl Pts',(94.6774190919,76.7803396540104,205.045723324001));
#26064=CARTESIAN_POINT('Ctrl Pts',(94.6279494551094,76.8136259651829,203.805110514219));
#26065=CARTESIAN_POINT('Ctrl Pts',(94.6116131950293,76.8254871376443,203.39159251221));
#26066=CARTESIAN_POINT('Ctrl Pts',(94.5878071200303,76.846762640332,202.771407418073));
#26067=CARTESIAN_POINT('Ctrl Pts',(94.579977356171,76.8543812940616,202.564692896978));
#26068=CARTESIAN_POINT('Ctrl Pts',(94.5687216025371,76.8682484451523,202.254685211554));
#26069=CARTESIAN_POINT('Ctrl Pts',(94.5650431963817,76.8732393054302,202.151351474201));
#26070=CARTESIAN_POINT('Ctrl Pts',(94.5598725495164,76.8824458559882,201.996442991466));
#26071=CARTESIAN_POINT('Ctrl Pts',(94.5582010160652,76.8857741808062,201.944813719824));
#26072=CARTESIAN_POINT('Ctrl Pts',(94.5559412686686,76.8919876567305,201.867463091344));
#26073=CARTESIAN_POINT('Ctrl Pts',(94.5552249685192,76.8942427868902,201.841685860449));
#26074=CARTESIAN_POINT('Ctrl Pts',(94.5543286074288,76.8984977281506,201.803113846285));
#26075=CARTESIAN_POINT('Ctrl Pts',(94.554056451558,76.9000460292448,201.790272515572));
#26076=CARTESIAN_POINT('Ctrl Pts',(94.5537773844895,76.902998912742,201.771088154141));
#26077=CARTESIAN_POINT('Ctrl Pts',(94.553703500895,76.9040778114373,201.764699617248));
#26078=CARTESIAN_POINT('Ctrl Pts',(94.5536883177333,76.9061537291684,201.75521495569));
#26079=CARTESIAN_POINT('Ctrl Pts',(94.5536973367198,76.9069141797371,201.75206293042));
#26080=CARTESIAN_POINT('Ctrl Pts',(94.5538111474632,76.9088856194884,201.745890870196));
#26081=CARTESIAN_POINT('Ctrl Pts',(94.5537483106129,76.9096547335994,201.741111962713));
#26082=CARTESIAN_POINT('Ctrl Pts',(94.5543840898181,76.912844378884,201.741111932358));
#26083=CARTESIAN_POINT('',(94.2048232844883,75.4756444900036,201.741111932485));
#26084=CARTESIAN_POINT('Ctrl Pts',(94.2048232844219,75.4756444900223,201.741111932358));
#26085=CARTESIAN_POINT('Ctrl Pts',(94.20572345773,75.4787698284284,201.741111962672));
#26086=CARTESIAN_POINT('Ctrl Pts',(94.2061325118859,75.4794241675821,201.745890870179));
#26087=CARTESIAN_POINT('Ctrl Pts',(94.2069368520303,75.4812276543486,201.752062930403));
#26088=CARTESIAN_POINT('Ctrl Pts',(94.207278098174,75.4819072994615,201.755214955672));
#26089=CARTESIAN_POINT('Ctrl Pts',(94.208245007057,75.4837443493165,201.764699617231));
#26090=CARTESIAN_POINT('Ctrl Pts',(94.2088061509609,75.4846687943932,201.771088154123));
#26091=CARTESIAN_POINT('Ctrl Pts',(94.2104102364897,75.4871636509014,201.790272515555));
#26092=CARTESIAN_POINT('Ctrl Pts',(94.2113630901064,75.4884140008851,201.803113846268));
#26093=CARTESIAN_POINT('Ctrl Pts',(94.2141135190867,75.4917819570548,201.841685860432));
#26094=CARTESIAN_POINT('Ctrl Pts',(94.2157855334549,75.4934561929679,201.867463091327));
#26095=CARTESIAN_POINT('Ctrl Pts',(94.2206465593263,75.4979377294053,201.944813719807));
#26096=CARTESIAN_POINT('Ctrl Pts',(94.2236599946165,75.5001265596694,201.996442991449));
#26097=CARTESIAN_POINT('Ctrl Pts',(94.2324814031209,75.505929913371,202.151351474185));
#26098=CARTESIAN_POINT('Ctrl Pts',(94.2380410940483,75.5086738512261,202.254685211539));
#26099=CARTESIAN_POINT('Ctrl Pts',(94.2544083679373,75.5158224325321,202.564692896964));
#26100=CARTESIAN_POINT('Ctrl Pts',(94.2648625664955,75.5189939966968,202.771407418059));
#26101=CARTESIAN_POINT('Ctrl Pts',(94.2957806900231,75.5269592875904,203.391592512198));
#26102=CARTESIAN_POINT('Ctrl Pts',(94.3157396417436,75.5299926111441,203.805110514209));
#26103=CARTESIAN_POINT('Ctrl Pts',(94.3749708212775,75.536840329118,205.045723392872));
#26104=CARTESIAN_POINT('Ctrl Pts',(94.4135109777832,75.5381062472439,205.872853797299));
#26105=CARTESIAN_POINT('Ctrl Pts',(94.4517292049929,75.5382477470648,206.699999961618));
#26106=CARTESIAN_POINT('',(79.2820076043964,62.8104109182795,201.741111932425));
#26107=CARTESIAN_POINT('Origin',(77.215862801455,80.368869783441,201.741111932358));
#26108=CARTESIAN_POINT('Ctrl Pts',(79.1801480918987,62.5769732298611,206.699999796081));
#26109=CARTESIAN_POINT('Ctrl Pts',(79.1864924085904,62.614659075419,205.872853767758));
#26110=CARTESIAN_POINT('Ctrl Pts',(79.1939985308776,62.6524797541957,205.045723525105));
#26111=CARTESIAN_POINT('Ctrl Pts',(79.2103717410791,62.7098082365092,203.805110800395));
#26112=CARTESIAN_POINT('Ctrl Pts',(79.2166052339168,62.7290080368152,203.391592818749));
#26113=CARTESIAN_POINT('Ctrl Pts',(79.2294846207187,62.7582191494274,202.771407717802));
#26114=CARTESIAN_POINT('Ctrl Pts',(79.2343114332871,62.7680184074779,202.564693188781));
#26115=CARTESIAN_POINT('Ctrl Pts',(79.2440225987803,62.783005387508,202.254685465399));
#26116=CARTESIAN_POINT('Ctrl Pts',(79.2476328247242,62.7880448952679,202.151351711356));
#26117=CARTESIAN_POINT('Ctrl Pts',(79.2547915027158,62.7958052813137,201.996443185338));
#26118=CARTESIAN_POINT('Ctrl Pts',(79.2574405860539,62.7984227159912,201.944813896416));
#26119=CARTESIAN_POINT('Ctrl Pts',(79.2626519789498,62.8024903940862,201.8674632292));
#26120=CARTESIAN_POINT('Ctrl Pts',(79.2645755011755,62.8038679447865,201.841685983602));
#26121=CARTESIAN_POINT('Ctrl Pts',(79.2683454016495,62.806034191599,201.803113937563));
#26122=CARTESIAN_POINT('Ctrl Pts',(79.2697338942366,62.8067710778536,201.790272595049));
#26123=CARTESIAN_POINT('Ctrl Pts',(79.2724561455209,62.8079481992474,201.771088210274));
#26124=CARTESIAN_POINT('Ctrl Pts',(79.2734594541819,62.8083515788154,201.764699663099));
#26125=CARTESIAN_POINT('Ctrl Pts',(79.2754291626288,62.809006954992,201.755214984094));
#26126=CARTESIAN_POINT('Ctrl Pts',(79.2761552123347,62.8092331645485,201.752062950592));
#26127=CARTESIAN_POINT('Ctrl Pts',(79.2780654103254,62.8097335953468,201.745890875593));
#26128=CARTESIAN_POINT('Ctrl Pts',(79.2787773537758,62.8100308058813,201.741111962317));
#26129=CARTESIAN_POINT('Ctrl Pts',(79.282007604389,62.8104109183449,201.741111932358));
#26130=CARTESIAN_POINT('Ctrl Pts',(77.8070980354593,62.6991535162783,201.741111932358));
#26131=CARTESIAN_POINT('Ctrl Pts',(77.8103484652123,62.6992622754927,201.741111963075));
#26132=CARTESIAN_POINT('Ctrl Pts',(77.8110973217177,62.6990752424435,201.745890864766));
#26133=CARTESIAN_POINT('Ctrl Pts',(77.8130610980324,62.6988670347964,201.752062910214));
#26134=CARTESIAN_POINT('Ctrl Pts',(77.8138129297545,62.6987523049169,201.755214927251));
#26135=CARTESIAN_POINT('Ctrl Pts',(77.8158588588416,62.6983998353157,201.764699571363));
#26136=CARTESIAN_POINT('Ctrl Pts',(77.8169114585462,62.698151535316,201.771088097973));
#26137=CARTESIAN_POINT('Ctrl Pts',(77.8197798875591,62.6973961234773,201.790272436059));
#26138=CARTESIAN_POINT('Ctrl Pts',(77.821263478527,62.6968758782787,201.803113754971));
#26139=CARTESIAN_POINT('Ctrl Pts',(77.8253164892923,62.6952997101382,201.841685737259));
#26140=CARTESIAN_POINT('Ctrl Pts',(77.8274254344019,62.6942263216229,201.867462953451));
#26141=CARTESIAN_POINT('Ctrl Pts',(77.8331896769943,62.690986511338,201.944813543195));
#26142=CARTESIAN_POINT('Ctrl Pts',(77.8362025123878,62.6887961330358,201.996442797555));
#26143=CARTESIAN_POINT('Ctrl Pts',(77.8444475817057,62.6821975801426,202.151351237008));
#26144=CARTESIAN_POINT('Ctrl Pts',(77.8487751077061,62.6777567617667,202.25468495767));
#26145=CARTESIAN_POINT('Ctrl Pts',(77.860631109217,62.664396421781,202.564692605138));
#26146=CARTESIAN_POINT('Ctrl Pts',(77.8668776431422,62.6554323033246,202.771407118306));
#26147=CARTESIAN_POINT('Ctrl Pts',(77.884006313118,62.6284843257675,203.391592205636));
#26148=CARTESIAN_POINT('Ctrl Pts',(77.8930581450468,62.6104372422142,203.805110228014));
#26149=CARTESIAN_POINT('Ctrl Pts',(77.9178720797775,62.5562147427134,205.045723192663));
#26150=CARTESIAN_POINT('Ctrl Pts',(77.9309841955656,62.5199487924835,205.872853690892));
#26151=CARTESIAN_POINT('Ctrl Pts',(77.9429274404634,62.4836418858484,206.699999961109));
#26152=CARTESIAN_POINT('Origin',(93.7337610429286,74.5888146207003,197.7));
#26153=CARTESIAN_POINT('Origin',(77.215862801455,80.368869783441,209.7));
#26154=CARTESIAN_POINT('',(82.4344268912437,95.2821721957428,209.7));
#26155=CARTESIAN_POINT('Origin',(92.1291652137568,75.1503056936523,207.5));
#26156=CARTESIAN_POINT('Origin',(77.215862801455,80.368869783441,209.7));
#26157=CARTESIAN_POINT('',(80.5848092391667,89.9964447584713,209.7));
#26158=CARTESIAN_POINT('Origin',(86.8434377764853,76.9999233457293,210.));
#26159=CARTESIAN_POINT('',(81.344473631984,92.1673685273507,210.));
#26160=CARTESIAN_POINT('Origin',(77.215862801455,80.368869783441,210.));
#26161=CARTESIAN_POINT('Origin',(77.215862801455,80.368869783441,209.7));
#26162=CARTESIAN_POINT('',(81.344473631984,92.1673685273507,209.7));
#26163=CARTESIAN_POINT('Origin',(77.215862801455,80.368869783441,209.4));
#26164=CARTESIAN_POINT('',(66.8117635085218,50.6366529487886,209.4));
#26165=CARTESIAN_POINT('Origin',(106.948079636107,69.9647704905078,208.1));
#26166=CARTESIAN_POINT('Origin',(77.215862801455,80.368869783441,194.026481344607));
#26167=CARTESIAN_POINT('',(69.7713582305978,49.7612015989078,194.026481344607));
#26168=CARTESIAN_POINT('',(84.6603673723122,110.976537967974,194.026481344607));
#26169=CARTESIAN_POINT('Origin',(77.215862801455,80.368869783441,194.026481344607));
#26170=CARTESIAN_POINT('Origin',(77.215862801455,80.368869783441,194.026481344607));
#26171=CARTESIAN_POINT('',(84.6012840027022,110.73361996651,193.776481344607));
#26172=CARTESIAN_POINT('Origin',(84.6012840027022,110.73361996651,194.026481344607));
#26173=CARTESIAN_POINT('Origin',(77.215862801455,80.368869783441,193.776481344607));
#26174=CARTESIAN_POINT('Origin',(77.215862801455,80.368869783441,195.376481344607));
#26175=CARTESIAN_POINT('',(72.5482766022668,61.1783476677416,195.126481344607));
#26176=CARTESIAN_POINT('Origin',(77.215862801455,80.368869783441,195.126481344607));
#26177=CARTESIAN_POINT('',(72.6073599718767,61.4212656692062,195.376481344607));
#26178=CARTESIAN_POINT('Origin',(72.5482766022668,61.1783476677416,195.376481344607));
#26179=CARTESIAN_POINT('Origin',(77.215862801455,80.368869783441,195.376481344607));
#26180=CARTESIAN_POINT('Origin',(77.215862801455,80.368869783441,197.021721166268));
#26181=CARTESIAN_POINT('',(73.0800269287566,63.3646096809226,197.021721166268));
#26182=CARTESIAN_POINT('',(81.3516986741534,97.3731298859594,197.021721166268));
#26183=CARTESIAN_POINT('Origin',(77.215862801455,80.368869783441,197.021721166268));
#26184=CARTESIAN_POINT('Origin',(77.215862801455,80.368869783441,197.021721166268));
#26185=CARTESIAN_POINT('',(81.3517414998324,97.3733059613665,197.031238072604));
#26186=CARTESIAN_POINT('Origin',(81.4107820437634,97.616047887424,197.021721166268));
#26187=CARTESIAN_POINT('Origin',(77.215862801455,80.368869783441,197.031238072604));
#26188=CARTESIAN_POINT('Origin',(87.0652037611821,97.7633458837792,207.276481344607));
#26189=CARTESIAN_POINT('',(86.0937896005589,96.188663441779,207.526481344607));
#26190=CARTESIAN_POINT('',(79.7412900434344,85.8911302979345,207.526481344607));
#26191=CARTESIAN_POINT('',(86.3065605834827,96.0574060274146,207.276481344607));
#26192=CARTESIAN_POINT('Origin',(86.0937896005589,96.188663441779,207.276481344607));
#26193=CARTESIAN_POINT('',(87.277974744106,97.6320884694148,207.276481344607));
#26194=CARTESIAN_POINT('Origin',(86.0937896005589,96.188663441779,207.276481344607));
#26195=CARTESIAN_POINT('Origin',(86.0937896005589,96.188663441779,207.276481344607));
#26196=CARTESIAN_POINT('Origin',(86.0937896005589,96.188663441779,207.276481344607));
#26197=CARTESIAN_POINT('Origin',(77.215862801455,80.368869783441,207.276481344607));
#26198=CARTESIAN_POINT('',(66.0612008874025,94.6747068168279,207.526481344607));
#26199=CARTESIAN_POINT('Origin',(77.215862801455,80.368869783441,207.526481344607));
#26200=CARTESIAN_POINT('Origin',(66.0612008874025,94.6747068168279,207.276481344607));
#26201=CARTESIAN_POINT('Origin',(85.9930972697295,96.0254382715203,202.246481277241));
#26202=CARTESIAN_POINT('',(85.7715372937515,95.6461913480132,197.285998193683));
#26203=CARTESIAN_POINT('',(85.7715371009377,95.6461914584938,197.285998250943));
#26204=CARTESIAN_POINT('',(86.1109957253458,95.7403933688821,197.526481344568));
#26205=CARTESIAN_POINT('Ctrl Pts',(85.7715374871662,95.646191237174,197.285998135919));
#26206=CARTESIAN_POINT('Ctrl Pts',(85.7725054328388,95.6456968118517,197.28708943318));
#26207=CARTESIAN_POINT('Ctrl Pts',(85.7727762193796,95.6455685834453,197.287529424681));
#26208=CARTESIAN_POINT('Ctrl Pts',(85.775448730368,95.6442257365666,197.290389369077));
#26209=CARTESIAN_POINT('Ctrl Pts',(85.7811525394671,95.6413790023973,197.296803694516));
#26210=CARTESIAN_POINT('Ctrl Pts',(85.8294132680089,95.6211973451069,197.348830628001));
#26211=CARTESIAN_POINT('Ctrl Pts',(85.8738913768775,95.6148707634768,197.390353160049));
#26212=CARTESIAN_POINT('Ctrl Pts',(85.9522239607591,95.6236167989524,197.452797942955));
#26213=CARTESIAN_POINT('Ctrl Pts',(85.9853072081226,95.6340261702735,197.475575268837));
#26214=CARTESIAN_POINT('Ctrl Pts',(86.0381104013451,95.6628199399351,197.50541610126));
#26215=CARTESIAN_POINT('Ctrl Pts',(86.0599824910312,95.67909256943,197.51545301994));
#26216=CARTESIAN_POINT('Ctrl Pts',(86.0912442094499,95.7119965209056,197.524679726807));
#26217=CARTESIAN_POINT('Ctrl Pts',(86.1018504288941,95.7256648117306,197.526481344743));
#26218=CARTESIAN_POINT('Ctrl Pts',(86.1109957247841,95.7403933692308,197.526481344607));
#26219=CARTESIAN_POINT('',(86.1113791955527,95.741012961473,197.526481344607));
#26220=CARTESIAN_POINT('',(86.1113791955527,95.741012961473,197.526481344607));
#26221=CARTESIAN_POINT('',(86.3065605834827,96.0574060274146,207.276481344607));
#26222=CARTESIAN_POINT('Origin',(86.6766969576459,97.1335683214121,183.174071706053));
#26223=CARTESIAN_POINT('',(86.8936178810123,97.009289147751,197.526481344607));
#26224=CARTESIAN_POINT('',(86.7995649337003,97.3512916790481,197.276481344607));
#26225=CARTESIAN_POINT('Ctrl Pts',(86.8936178810123,97.0092891477511,197.526481344607));
#26226=CARTESIAN_POINT('Ctrl Pts',(86.8938783775809,97.0097438269587,197.526481344607));
#26227=CARTESIAN_POINT('Ctrl Pts',(86.8941375763002,97.0101995550636,197.526479697129));
#26228=CARTESIAN_POINT('Ctrl Pts',(86.9059119225634,97.0310539697099,197.526329043289));
#26229=CARTESIAN_POINT('Ctrl Pts',(86.914296385724,97.0525943485027,197.522897090167));
#26230=CARTESIAN_POINT('Ctrl Pts',(86.9257598377503,97.0997764576947,197.509425478113));
#26231=CARTESIAN_POINT('Ctrl Pts',(86.9276623879705,97.1246972156251,197.49872862438));
#26232=CARTESIAN_POINT('Ctrl Pts',(86.9243822484398,97.180003725259,197.468545557741));
#26233=CARTESIAN_POINT('Ctrl Pts',(86.9166406619662,97.2092432027731,197.447428878785));
#26234=CARTESIAN_POINT('Ctrl Pts',(86.8941169849787,97.259932057604,197.403006214921));
#26235=CARTESIAN_POINT('Ctrl Pts',(86.8794821770795,97.2819696349757,197.37953436841));
#26236=CARTESIAN_POINT('Ctrl Pts',(86.8446722048286,97.3206341661874,197.330483552621));
#26237=CARTESIAN_POINT('Ctrl Pts',(86.8240336652295,97.3372030242998,197.304533630732));
#26238=CARTESIAN_POINT('Ctrl Pts',(86.8008698123469,97.3505514194756,197.277971923767));
#26239=CARTESIAN_POINT('Ctrl Pts',(86.8002182010604,97.3509230202178,197.277226632397));
#26240=CARTESIAN_POINT('Ctrl Pts',(86.7995649337003,97.3512916790481,197.276481344607));
#26241=CARTESIAN_POINT('',(86.7995649337003,97.3512916790481,183.174071706053));
#26242=CARTESIAN_POINT('',(86.8894679405697,97.0023109070477,197.526481344607));
#26243=CARTESIAN_POINT('',(86.8894679405697,97.0023109070477,197.526481344607));
#26244=CARTESIAN_POINT('Origin',(86.6766969576459,97.1335683214121,197.526481344607));
#26245=CARTESIAN_POINT('Origin',(77.215862801455,80.368869783441,207.276481344607));
#26246=CARTESIAN_POINT('Origin',(77.215862801455,80.368869783441,207.526481344607));
#26247=CARTESIAN_POINT('Origin',(77.215862801455,80.368869783441,207.276481344607));
#26248=CARTESIAN_POINT('Origin',(66.0612008874025,94.6747068168279,207.276481344607));
#26249=CARTESIAN_POINT('',(65.8706178185259,94.512910358716,207.276481344607));
#26250=CARTESIAN_POINT('Origin',(66.0612008874025,94.6747068168279,207.276481344607));
#26251=CARTESIAN_POINT('Origin',(66.0612008874025,94.6747068168279,207.276481344607));
#26252=CARTESIAN_POINT('Origin',(77.215862801455,80.368869783441,197.276481344607));
#26253=CARTESIAN_POINT('',(87.0302049776637,94.8697252003878,197.285998170767));
#26254=CARTESIAN_POINT('',(86.9620814661663,95.2153625964141,197.526481344568));
#26255=CARTESIAN_POINT('Ctrl Pts',(87.0302047491998,94.8697253476385,197.285998010414));
#26256=CARTESIAN_POINT('Ctrl Pts',(87.0293873488746,94.8703254048265,197.287016105511));
#26257=CARTESIAN_POINT('Ctrl Pts',(87.0293554761683,94.8703809253921,197.287632834136));
#26258=CARTESIAN_POINT('Ctrl Pts',(87.0282421949799,94.8711981752271,197.288758182633));
#26259=CARTESIAN_POINT('Ctrl Pts',(87.0274485389422,94.8717814515778,197.289656234906));
#26260=CARTESIAN_POINT('Ctrl Pts',(87.0076896512662,94.8869284991216,197.313936094399));
#26261=CARTESIAN_POINT('Ctrl Pts',(86.9916554589569,94.9030932672712,197.336722197331));
#26262=CARTESIAN_POINT('Ctrl Pts',(86.9533411021071,94.953758427131,197.396368011346));
#26263=CARTESIAN_POINT('Ctrl Pts',(86.9367358693936,94.9912035179937,197.430388733357));
#26264=CARTESIAN_POINT('Ctrl Pts',(86.9232850558868,95.0616415164893,197.47902078915));
#26265=CARTESIAN_POINT('Ctrl Pts',(86.9229006039806,95.0928025207568,197.495729267709));
#26266=CARTESIAN_POINT('Ctrl Pts',(86.9318852326942,95.1474151109197,197.516701595193));
#26267=CARTESIAN_POINT('Ctrl Pts',(86.9394044252834,95.171765230652,197.523029647908));
#26268=CARTESIAN_POINT('Ctrl Pts',(86.9543584616972,95.2020873466914,197.526129019956));
#26269=CARTESIAN_POINT('Ctrl Pts',(86.9580752868692,95.2088258280812,197.5264813447));
#26270=CARTESIAN_POINT('Ctrl Pts',(86.9620814697059,95.2153625942447,197.526481344607));
#26271=CARTESIAN_POINT('Origin',(77.215862801455,80.368869783441,197.526481344607));
#26272=CARTESIAN_POINT('Origin',(77.215862801455,80.368869783441,197.285998250943));
#26273=CARTESIAN_POINT('Origin',(77.215862801455,80.368869783441,197.276481344607));
#26274=CARTESIAN_POINT('',(87.744926219196,96.4841210549909,197.526481344607));
#26275=CARTESIAN_POINT('',(88.0927703883544,96.553519342392,197.276481344607));
#26276=CARTESIAN_POINT('Ctrl Pts',(87.744926219196,96.4841210549908,197.526481344607));
#26277=CARTESIAN_POINT('Ctrl Pts',(87.7452156792141,96.4845578667829,197.526481344607));
#26278=CARTESIAN_POINT('Ctrl Pts',(87.745506658949,96.484993989329,197.526479697129));
#26279=CARTESIAN_POINT('Ctrl Pts',(87.7588610072407,96.5048737081865,197.526329043289));
#26280=CARTESIAN_POINT('Ctrl Pts',(87.7743493927896,96.5220317108126,197.522897090168));
#26281=CARTESIAN_POINT('Ctrl Pts',(87.8113719962568,96.5534465002068,197.509425478114));
#26282=CARTESIAN_POINT('Ctrl Pts',(87.8327897428621,96.5663284256653,197.49872862438));
#26283=CARTESIAN_POINT('Ctrl Pts',(87.8836882989136,96.5882123539018,197.468545557742));
#26284=CARTESIAN_POINT('Ctrl Pts',(87.9132928417027,96.5944131806742,197.447428878786));
#26285=CARTESIAN_POINT('Ctrl Pts',(87.9686989911511,96.5970274936707,197.403006214922));
#26286=CARTESIAN_POINT('Ctrl Pts',(87.9949601815994,96.5938365228299,197.379534368411));
#26287=CARTESIAN_POINT('Ctrl Pts',(88.0451330397623,96.580075547367,197.330483552623));
#26288=CARTESIAN_POINT('Ctrl Pts',(88.0692006987673,96.5690653627259,197.304533630731));
#26289=CARTESIAN_POINT('Ctrl Pts',(88.0915233437827,96.554353352199,197.27797192377));
#26290=CARTESIAN_POINT('Ctrl Pts',(88.0921478091168,96.5539377473013,197.277226632396));
#26291=CARTESIAN_POINT('Ctrl Pts',(88.0927703883544,96.5535193423919,197.276481344607));
#26292=CARTESIAN_POINT('Origin',(77.215862801455,80.368869783441,197.276481344607));
#26293=CARTESIAN_POINT('Origin',(77.215862801455,80.368869783441,197.526481344607));
#26294=CARTESIAN_POINT('Origin',(64.8042619416421,96.1552786690737,207.276481344607));
#26295=CARTESIAN_POINT('',(64.6136788727654,95.9934822109618,207.276481344607));
#26296=CARTESIAN_POINT('',(88.001300134864,68.8310542744068,207.526481344607));
#26297=CARTESIAN_POINT('Origin',(66.1853223820777,94.5285011270022,202.246481276341));
#26298=CARTESIAN_POINT('',(66.1112139395638,94.2295076956275,197.526481344607));
#26299=CARTESIAN_POINT('',(66.1112139395638,94.2295076956275,197.526481344607));
#26300=CARTESIAN_POINT('',(66.1116408285149,94.2290061991774,197.526481344578));
#26301=CARTESIAN_POINT('',(66.1116408097593,94.2290062155739,197.52648134452));
#26302=CARTESIAN_POINT('',(66.4614031347772,94.1868912572728,197.285998169697));
#26303=CARTESIAN_POINT('Ctrl Pts',(66.1116408313988,94.2290062016389,197.526481344607));
#26304=CARTESIAN_POINT('Ctrl Pts',(66.1169211525317,94.2228196133348,197.526481344688));
#26305=CARTESIAN_POINT('Ctrl Pts',(66.1225164472751,94.2168744591204,197.526084798852));
#26306=CARTESIAN_POINT('Ctrl Pts',(66.1472603113197,94.1930214631972,197.522744043761));
#26307=CARTESIAN_POINT('Ctrl Pts',(66.1682407124789,94.1784248076749,197.516246088138));
#26308=CARTESIAN_POINT('Ctrl Pts',(66.2177375812335,94.1532020157617,197.494874084349));
#26309=CARTESIAN_POINT('Ctrl Pts',(66.2477024906526,94.1440934241378,197.477895158506));
#26310=CARTESIAN_POINT('Ctrl Pts',(66.3192752562298,94.1356134414265,197.428597050384));
#26311=CARTESIAN_POINT('Ctrl Pts',(66.3601923972269,94.1402155954496,197.394186199542));
#26312=CARTESIAN_POINT('Ctrl Pts',(66.432503312338,94.1660665527557,197.32179389136));
#26313=CARTESIAN_POINT('Ctrl Pts',(66.454375282936,94.1820035053602,197.294649845323));
#26314=CARTESIAN_POINT('Ctrl Pts',(66.4584424176479,94.1848017482204,197.289840338499));
#26315=CARTESIAN_POINT('Ctrl Pts',(66.4593281118165,94.1854321505868,197.28882852111));
#26316=CARTESIAN_POINT('Ctrl Pts',(66.4605216743804,94.1862901108438,197.287634889492));
#26317=CARTESIAN_POINT('Ctrl Pts',(66.460580587625,94.186300146126,197.287014717403));
#26318=CARTESIAN_POINT('Ctrl Pts',(66.4614029209132,94.1868910829801,197.285998007206));
#26319=CARTESIAN_POINT('',(66.35154481532,94.3164511783277,201.74111193235));
#26320=CARTESIAN_POINT('Origin',(87.2697224402081,95.237894233865,202.246481277241));
#26321=CARTESIAN_POINT('',(87.1194741085686,95.0142415830358,201.741111932351));
#26322=CARTESIAN_POINT('',(86.9624631272481,95.2159833040156,197.526481344607));
#26323=CARTESIAN_POINT('',(86.9624631272481,95.2159833040156,197.526481344607));
#26324=CARTESIAN_POINT('',(86.9620814785655,95.2153626241862,197.526481344489));
#26325=CARTESIAN_POINT('Origin',(87.953322855189,96.3460238352259,183.174071706053));
#26326=CARTESIAN_POINT('',(87.7405518722651,96.4772812495903,207.276481344607));
#26327=CARTESIAN_POINT('',(88.0927703883544,96.553519342392,207.276481344607));
#26328=CARTESIAN_POINT('Origin',(87.953322855189,96.3460238352259,207.276481344607));
#26329=CARTESIAN_POINT('',(88.0927703883544,96.553519342392,183.174071706053));
#26330=CARTESIAN_POINT('',(87.7405518722651,96.4772812495903,197.526481344607));
#26331=CARTESIAN_POINT('Origin',(87.953322855189,96.3460238352259,197.526481344607));
#26332=CARTESIAN_POINT('',(87.7405518722651,96.4772812495903,197.526481344607));
#26333=CARTESIAN_POINT('Origin',(65.3426635064322,95.5210854135286,183.174071706053));
#26334=CARTESIAN_POINT('',(65.1520804375556,95.3592889554166,197.526481344607));
#26335=CARTESIAN_POINT('',(65.1468869158002,95.3656134657036,197.526481344607));
#26336=CARTESIAN_POINT('Origin',(65.3426635064322,95.5210854135286,197.526481344607));
#26337=CARTESIAN_POINT('',(65.1520804375556,95.3592889554166,197.526481344607));
#26338=CARTESIAN_POINT('',(65.1884661129904,95.7178674346986,197.276481344607));
#26339=CARTESIAN_POINT('',(65.1884661129904,95.7178674346986,183.174071706053));
#26340=CARTESIAN_POINT('Ctrl Pts',(65.1884661129904,95.7178674346985,197.276481344607));
#26341=CARTESIAN_POINT('Ctrl Pts',(65.1878756789987,95.7174047736182,197.277226632395));
#26342=CARTESIAN_POINT('Ctrl Pts',(65.1872873244521,95.7169394529637,197.277971923769));
#26343=CARTESIAN_POINT('Ctrl Pts',(65.1663929788226,95.7002610221315,197.304533630727));
#26344=CARTESIAN_POINT('Ctrl Pts',(65.1484793144624,95.6807782860578,197.330483552621));
#26345=CARTESIAN_POINT('Ctrl Pts',(65.1198763396659,95.6373208358935,197.37953436841));
#26346=CARTESIAN_POINT('Ctrl Pts',(65.1087201860209,95.6133339091515,197.403006214922));
#26347=CARTESIAN_POINT('Ctrl Pts',(65.0940712628922,95.5598354504791,197.447428878785));
#26348=CARTESIAN_POINT('Ctrl Pts',(65.0908125131871,95.5297645383416,197.468545557742));
#26349=CARTESIAN_POINT('Ctrl Pts',(65.0958825740711,95.4745933157176,197.49872862438));
#26350=CARTESIAN_POINT('Ctrl Pts',(65.1015092658451,95.4502416378935,197.509425478113));
#26351=CARTESIAN_POINT('Ctrl Pts',(65.1199342711905,95.4053185776885,197.522897090168));
#26352=CARTESIAN_POINT('Ctrl Pts',(65.131461144181,95.3852831505632,197.526329043289));
#26353=CARTESIAN_POINT('Ctrl Pts',(65.1462362842778,95.3664354166072,197.526479697129));
#26354=CARTESIAN_POINT('Ctrl Pts',(65.1465610373146,95.3660238251271,197.526481344607));
#26355=CARTESIAN_POINT('Ctrl Pts',(65.1468869158002,95.3656134657036,197.526481344607));
#26356=CARTESIAN_POINT('Origin',(77.215862801455,80.368869783441,197.276481344607));
#26357=CARTESIAN_POINT('',(65.3491255130522,93.5820326593704,197.526481344555));
#26358=CARTESIAN_POINT('',(65.3337218174719,93.230084572225,197.285998194441));
#26359=CARTESIAN_POINT('Ctrl Pts',(65.3491255125137,93.5820326589161,197.526481344607));
#26360=CARTESIAN_POINT('Ctrl Pts',(65.3602746962636,93.5688145431561,197.526481344716));
#26361=CARTESIAN_POINT('Ctrl Pts',(65.36997193769,93.554539724584,197.524688976763));
#26362=CARTESIAN_POINT('Ctrl Pts',(65.39158902819,93.5146913614094,197.515495497821));
#26363=CARTESIAN_POINT('Ctrl Pts',(65.4003109763584,93.4888725096656,197.505476486175));
#26364=CARTESIAN_POINT('Ctrl Pts',(65.4113928007713,93.4297827815416,197.475678704812));
#26365=CARTESIAN_POINT('Ctrl Pts',(65.4110836642222,93.3951188265962,197.452930521194));
#26366=CARTESIAN_POINT('Ctrl Pts',(65.3952406789993,93.3179425315011,197.390550112667));
#26367=CARTESIAN_POINT('Ctrl Pts',(65.3755108879767,93.2775983899897,197.349058772659));
#26368=CARTESIAN_POINT('Ctrl Pts',(65.341353172853,93.2378215388855,197.296918842359));
#26369=CARTESIAN_POINT('Ctrl Pts',(65.3368138008746,93.2332094505631,197.290407199789));
#26370=CARTESIAN_POINT('Ctrl Pts',(65.3346982702197,93.2310710756822,197.287528959007));
#26371=CARTESIAN_POINT('Ctrl Pts',(65.3344917686414,93.2308525241048,197.287089779763));
#26372=CARTESIAN_POINT('Ctrl Pts',(65.3337219804242,93.2300847198161,197.285998137443));
#26373=CARTESIAN_POINT('Origin',(77.215862801455,80.368869783441,197.285998250943));
#26374=CARTESIAN_POINT('Origin',(77.215862801455,80.368869783441,197.526481344607));
#26375=CARTESIAN_POINT('Origin',(87.953322855189,96.3460238352259,207.276481344607));
#26376=CARTESIAN_POINT('',(87.953322855189,96.3460238352259,207.526481344607));
#26377=CARTESIAN_POINT('Origin',(87.953322855189,96.3460238352259,207.276481344607));
#26378=CARTESIAN_POINT('Origin',(87.953322855189,96.3460238352259,207.276481344607));
#26379=CARTESIAN_POINT('Origin',(77.215862801455,80.368869783441,197.276481344607));
#26380=CARTESIAN_POINT('',(64.3841861492998,94.7184542476175,197.526481344607));
#26381=CARTESIAN_POINT('Origin',(77.215862801455,80.368869783441,197.526481344607));
#26382=CARTESIAN_POINT('',(64.0298626660881,94.7347808380907,197.276481344607));
#26383=CARTESIAN_POINT('Origin',(77.215862801455,80.368869783441,197.276481344607));
#26384=CARTESIAN_POINT('Ctrl Pts',(64.0298626660881,94.7347808380907,197.276481344607));
#26385=CARTESIAN_POINT('Ctrl Pts',(64.0304152834259,94.73528806748,197.277226632396));
#26386=CARTESIAN_POINT('Ctrl Pts',(64.030970186294,94.7357928121606,197.277971923767));
#26387=CARTESIAN_POINT('Ctrl Pts',(64.050827920147,94.7536929277923,197.304533630741));
#26388=CARTESIAN_POINT('Ctrl Pts',(64.0729672526987,94.7681955596412,197.330483552619));
#26389=CARTESIAN_POINT('Ctrl Pts',(64.1205017521378,94.7893415168146,197.379534368405));
#26390=CARTESIAN_POINT('Ctrl Pts',(64.1459849761886,94.796443467996,197.403006214916));
#26391=CARTESIAN_POINT('Ctrl Pts',(64.2011546284904,94.8021867679137,197.44742887878));
#26392=CARTESIAN_POINT('Ctrl Pts',(64.2313548721284,94.8005061458102,197.468545557738));
#26393=CARTESIAN_POINT('Ctrl Pts',(64.2849644912409,94.7865212231472,197.498728624377));
#26394=CARTESIAN_POINT('Ctrl Pts',(64.3080751589899,94.7770048735645,197.509425478111));
#26395=CARTESIAN_POINT('Ctrl Pts',(64.3493990161624,94.7515117178442,197.522897090166));
#26396=CARTESIAN_POINT('Ctrl Pts',(64.3672904066541,94.7368766473865,197.526329043289));
#26397=CARTESIAN_POINT('Ctrl Pts',(64.3834810958367,94.7192300209656,197.526479697129));
#26398=CARTESIAN_POINT('Ctrl Pts',(64.383834321995,94.7188425892111,197.526481344607));
#26399=CARTESIAN_POINT('Ctrl Pts',(64.3841861492998,94.7184542476174,197.526481344607));
#26400=CARTESIAN_POINT('Origin',(65.0415552428384,93.5580402355824,202.246481278135));
#26401=CARTESIAN_POINT('',(65.3337216550388,93.2300844250878,197.285998250943));
#26402=CARTESIAN_POINT('',(65.3486095562104,93.5826423840931,197.526481344607));
#26403=CARTESIAN_POINT('',(65.3486095562104,93.5826423840931,197.526481344607));
#26404=CARTESIAN_POINT('',(65.1080190161996,93.8660384731857,207.276481344607));
#26405=CARTESIAN_POINT('Origin',(77.215862801455,80.368869783441,207.276481344607));
#26406=CARTESIAN_POINT('',(95.0048109024016,76.8140447378918,207.526481344607));
#26407=CARTESIAN_POINT('Origin',(95.0048109024016,76.8140447378918,207.276481344607));
#26408=CARTESIAN_POINT('Origin',(77.215862801455,80.368869783441,207.526481344607));
#26409=CARTESIAN_POINT('Origin',(88.3891501308591,97.0525088614501,207.276481344607));
#26410=CARTESIAN_POINT('',(81.0179159409774,85.1035858117482,207.526481344607));
#26411=CARTESIAN_POINT('',(88.1763791479352,97.1837662758145,207.276481344607));
#26412=CARTESIAN_POINT('Origin',(77.215862801455,80.368869783441,207.276481344607));
#26413=CARTESIAN_POINT('Origin',(77.215862801455,80.368869783441,207.276481344607));
#26414=CARTESIAN_POINT('Origin',(77.215862801455,80.368869783441,207.526481344607));
#26415=CARTESIAN_POINT('Origin',(64.1989139498749,94.5506024912362,183.174071706053));
#26416=CARTESIAN_POINT('',(64.0298626660881,94.7347808380907,207.276481344607));
#26417=CARTESIAN_POINT('',(64.3894970187515,94.7123989493481,207.276481344607));
#26418=CARTESIAN_POINT('Origin',(64.1989139498749,94.5506024912362,207.276481344607));
#26419=CARTESIAN_POINT('',(64.3894970187515,94.7123989493481,197.526481344607));
#26420=CARTESIAN_POINT('',(64.3894970187515,94.7123989493481,197.526481344607));
#26421=CARTESIAN_POINT('Origin',(64.1989139498749,94.5506024912362,197.526481344607));
#26422=CARTESIAN_POINT('',(64.0298626660881,94.7347808380907,183.174071706053));
#26423=CARTESIAN_POINT('Origin',(95.0048109024016,76.8140447378918,207.276481344607));
#26424=CARTESIAN_POINT('',(94.9457275327917,76.5711267364272,207.276481344607));
#26425=CARTESIAN_POINT('Origin',(95.0048109024016,76.8140447378918,207.276481344607));
#26426=CARTESIAN_POINT('Origin',(95.0048109024016,76.8140447378918,207.276481344607));
#26427=CARTESIAN_POINT('Origin',(64.1989139498749,94.5506024912362,207.276481344607));
#26428=CARTESIAN_POINT('',(64.1989139498749,94.5506024912362,207.526481344607));
#26429=CARTESIAN_POINT('Origin',(64.1989139498749,94.5506024912362,207.276481344607));
#26430=CARTESIAN_POINT('Origin',(64.1989139498749,94.5506024912362,207.276481344607));
#26431=CARTESIAN_POINT('Origin',(63.719093831661,95.1157915670977,207.276481344607));
#26432=CARTESIAN_POINT('',(86.8578017216042,67.8602755257353,207.526481344607));
#26433=CARTESIAN_POINT('',(63.9096769005376,95.2775880252097,207.276481344607));
#26434=CARTESIAN_POINT('Origin',(77.215862801455,80.368869783441,207.276481344607));
#26435=CARTESIAN_POINT('Origin',(77.215862801455,80.368869783441,207.526481344607));
#26436=CARTESIAN_POINT('Origin',(94.8184588991746,76.8593694837389,202.246481277241));
#26437=CARTESIAN_POINT('',(94.3893078434365,76.95289179822,197.285998193683));
#26438=CARTESIAN_POINT('',(94.389307888928,76.9528920157415,197.285998250943));
#26439=CARTESIAN_POINT('',(94.5837977134794,76.6591576701982,197.526481344568));
#26440=CARTESIAN_POINT('Ctrl Pts',(94.3893077977898,76.9528915800162,197.285998135919));
#26441=CARTESIAN_POINT('Ctrl Pts',(94.3891366830531,76.9518182233094,197.287089433018));
#26442=CARTESIAN_POINT('Ctrl Pts',(94.3890984083501,76.9515210657439,197.287529424903));
#26443=CARTESIAN_POINT('Ctrl Pts',(94.3886471375595,76.9485644021981,197.290389360712));
#26444=CARTESIAN_POINT('Ctrl Pts',(94.3877023133716,76.9422601127003,197.296803640722));
#26445=CARTESIAN_POINT('Ctrl Pts',(94.3834217828299,76.8901250153594,197.348830521281));
#26446=CARTESIAN_POINT('Ctrl Pts',(94.3911493204423,76.8458687886726,197.390353067837));
#26447=CARTESIAN_POINT('Ctrl Pts',(94.423673374515,76.7740727220947,197.45279788084));
#26448=CARTESIAN_POINT('Ctrl Pts',(94.4437965561254,76.7458253439581,197.475575220366));
#26449=CARTESIAN_POINT('Ctrl Pts',(94.4874981390143,76.7045042673687,197.505416072974));
#26450=CARTESIAN_POINT('Ctrl Pts',(94.5097331760758,76.6887311845888,197.51545300005));
#26451=CARTESIAN_POINT('Ctrl Pts',(94.5506871134101,76.6691673834714,197.524679722475));
#26452=CARTESIAN_POINT('Ctrl Pts',(94.5669639509563,76.6633039945062,197.526481344743));
#26453=CARTESIAN_POINT('Ctrl Pts',(94.5837977136375,76.6591576708401,197.526481344607));
#26454=CARTESIAN_POINT('',(94.5845054798612,76.6589844329993,197.526481344607));
#26455=CARTESIAN_POINT('',(94.5845054798612,76.6589844329993,197.526481344607));
#26456=CARTESIAN_POINT('',(94.9457275327917,76.5711267364272,207.276481344607));
#26457=CARTESIAN_POINT('Origin',(96.4901086410159,76.4527854045269,207.276481344607));
#26458=CARTESIAN_POINT('',(96.4310252714059,76.2098674030624,207.276481344607));
#26459=CARTESIAN_POINT('',(96.3407170245198,76.4891209582564,207.526481344607));
#26460=CARTESIAN_POINT('Origin',(96.0835971249419,76.5516585634122,183.174071706053));
#26461=CARTESIAN_POINT('',(96.0324328587475,76.3069501290158,197.526481344607));
#26462=CARTESIAN_POINT('',(96.3286326356366,76.5020843917236,197.276481344607));
#26463=CARTESIAN_POINT('Ctrl Pts',(96.0324328587475,76.3069501290157,197.526481344607));
#26464=CARTESIAN_POINT('Ctrl Pts',(96.0329457822375,76.3068428856588,197.526481344607));
#26465=CARTESIAN_POINT('Ctrl Pts',(96.0334593022307,76.306737200757,197.526479697129));
#26466=CARTESIAN_POINT('Ctrl Pts',(96.0569315022667,76.3019835005518,197.526329043289));
#26467=CARTESIAN_POINT('Ctrl Pts',(96.0800085614862,76.3006657453395,197.522897090167));
#26468=CARTESIAN_POINT('Ctrl Pts',(96.1284238153765,76.3043434281616,197.509425478113));
#26469=CARTESIAN_POINT('Ctrl Pts',(96.1527127849481,76.3102349330904,197.498728624379));
#26470=CARTESIAN_POINT('Ctrl Pts',(96.2042987824697,76.3304451825418,197.468545557741));
#26471=CARTESIAN_POINT('Ctrl Pts',(96.2297148963087,76.3468433642625,197.447428878784));
#26472=CARTESIAN_POINT('Ctrl Pts',(96.2709626630343,76.3839283716008,197.403006214921));
#26473=CARTESIAN_POINT('Ctrl Pts',(96.2873992402467,76.4046568869407,197.379534368409));
#26474=CARTESIAN_POINT('Ctrl Pts',(96.3134145216056,76.4497111351057,197.330483552621));
#26475=CARTESIAN_POINT('Ctrl Pts',(96.3227947826065,76.4744596114168,197.304533630737));
#26476=CARTESIAN_POINT('Ctrl Pts',(96.3283318366233,76.5006146255939,197.277971923768));
#26477=CARTESIAN_POINT('Ctrl Pts',(96.3284838909699,76.5013491757008,197.277226632396));
#26478=CARTESIAN_POINT('Ctrl Pts',(96.3286326356366,76.5020843917236,197.276481344607));
#26479=CARTESIAN_POINT('',(96.3286326356366,76.5020843917236,183.174071706053));
#26480=CARTESIAN_POINT('',(96.0245137553319,76.3087405619477,197.526481344607));
#26481=CARTESIAN_POINT('',(96.0245137553319,76.3087405619477,197.526481344607));
#26482=CARTESIAN_POINT('Origin',(96.0835971249419,76.5516585634122,197.526481344607));
#26483=CARTESIAN_POINT('Origin',(77.215862801455,80.368869783441,207.276481344607));
#26484=CARTESIAN_POINT('',(58.9003582657663,73.6761652775505,207.276481344607));
#26485=CARTESIAN_POINT('',(59.1351724264803,73.7619691814722,207.526481344607));
#26486=CARTESIAN_POINT('Origin',(59.1351724264803,73.7619691814722,207.276481344607));
#26487=CARTESIAN_POINT('Origin',(77.215862801455,80.368869783441,207.526481344607));
#26488=CARTESIAN_POINT('Origin',(77.215862801455,80.368869783441,207.276481344607));
#26489=CARTESIAN_POINT('Origin',(77.215862801455,80.368869783441,197.276481344607));
#26490=CARTESIAN_POINT('',(94.0397943586528,75.5158864604089,197.285998170767));
#26491=CARTESIAN_POINT('',(94.3474637336519,75.6874835992026,197.526481344568));
#26492=CARTESIAN_POINT('Ctrl Pts',(94.0397944280951,75.5158867231863,197.285998010414));
#26493=CARTESIAN_POINT('Ctrl Pts',(94.0401125259821,75.5168495455053,197.287016106087));
#26494=CARTESIAN_POINT('Ctrl Pts',(94.0401554804701,75.5168970170074,197.287632833281));
#26495=CARTESIAN_POINT('Ctrl Pts',(94.0405887095143,75.518208357421,197.288758185983));
#26496=CARTESIAN_POINT('Ctrl Pts',(94.0408981874299,75.5191434185213,197.289656246106));
#26497=CARTESIAN_POINT('Ctrl Pts',(94.0491981798594,75.54261627962,197.313936475957));
#26498=CARTESIAN_POINT('Ctrl Pts',(94.0596171630581,75.5628612000245,197.336722933864));
#26499=CARTESIAN_POINT('Ctrl Pts',(94.095963205002,75.6149568033014,197.396368929828));
#26500=CARTESIAN_POINT('Ctrl Pts',(94.1264443408684,75.6423203109527,197.430389486829));
#26501=CARTESIAN_POINT('Ctrl Pts',(94.189278308267,75.6768790524282,197.479021261726));
#26502=CARTESIAN_POINT('Ctrl Pts',(94.2187953499103,75.6868738596624,197.49572962646));
#26503=CARTESIAN_POINT('Ctrl Pts',(94.273511348843,75.6952050320096,197.516701785659));
#26504=CARTESIAN_POINT('Ctrl Pts',(94.2989932171594,75.6955783896931,197.52302976678));
#26505=CARTESIAN_POINT('Ctrl Pts',(94.3324520692234,75.6907262606351,197.526129038087));
#26506=CARTESIAN_POINT('Ctrl Pts',(94.3400091118565,75.6892736835662,197.5264813447));
#26507=CARTESIAN_POINT('Ctrl Pts',(94.3474637326825,75.6874835951658,197.526481344607));
#26508=CARTESIAN_POINT('Origin',(77.215862801455,80.368869783441,197.526481344607));
#26509=CARTESIAN_POINT('Origin',(77.215862801455,80.368869783441,197.285998250943));
#26510=CARTESIAN_POINT('Origin',(77.215862801455,80.368869783441,197.276481344607));
#26511=CARTESIAN_POINT('',(95.7960370659294,75.3350219210433,197.526481344607));
#26512=CARTESIAN_POINT('',(95.969528519046,75.0256477074975,197.276481344607));
#26513=CARTESIAN_POINT('Ctrl Pts',(95.7960370659294,75.3350219210434,197.526481344607));
#26514=CARTESIAN_POINT('Ctrl Pts',(95.7965419466967,75.3348816104736,197.526481344607));
#26515=CARTESIAN_POINT('Ctrl Pts',(95.7970466415705,75.3347396415787,197.526479697129));
#26516=CARTESIAN_POINT('Ctrl Pts',(95.8200800983042,75.3281820725845,197.526329043289));
#26517=CARTESIAN_POINT('Ctrl Pts',(95.8411845028582,75.3187538569821,197.522897090167));
#26518=CARTESIAN_POINT('Ctrl Pts',(95.8825023566668,75.2932509725011,197.509425478112));
#26519=CARTESIAN_POINT('Ctrl Pts',(95.9013722434987,75.2768622189142,197.498728624378));
#26520=CARTESIAN_POINT('Ctrl Pts',(95.9379136148588,75.235217321239,197.468545557739));
#26521=CARTESIAN_POINT('Ctrl Pts',(95.9529592583993,75.2089778887585,197.447428878781));
#26522=CARTESIAN_POINT('Ctrl Pts',(95.972567059581,75.1570913764279,197.403006214918));
#26523=CARTESIAN_POINT('Ctrl Pts',(95.97764742011,75.1311294359093,197.379534368408));
#26524=CARTESIAN_POINT('Ctrl Pts',(95.9800642205536,75.0791598369372,197.330483552621));
#26525=CARTESIAN_POINT('Ctrl Pts',(95.9770302283516,75.0528677988418,197.304533630734));
#26526=CARTESIAN_POINT('Ctrl Pts',(95.9699363515425,75.0270914405678,197.277971923769));
#26527=CARTESIAN_POINT('Ctrl Pts',(95.9697340581972,75.026369109767,197.277226632397));
#26528=CARTESIAN_POINT('Ctrl Pts',(95.9695285190461,75.0256477074975,197.276481344607));
#26529=CARTESIAN_POINT('Origin',(77.215862801455,80.368869783441,197.276481344607));
#26530=CARTESIAN_POINT('Origin',(77.215862801455,80.368869783441,197.526481344607));
#26531=CARTESIAN_POINT('Origin',(59.1351724264803,73.7619691814722,207.276481344607));
#26532=CARTESIAN_POINT('',(59.2301565951581,73.5307160567353,207.276481344607));
#26533=CARTESIAN_POINT('Origin',(59.1351724264803,73.7619691814722,207.276481344607));
#26534=CARTESIAN_POINT('Origin',(59.1351724264803,73.7619691814722,207.276481344607));
#26535=CARTESIAN_POINT('Origin',(58.3694473018174,73.4474576933157,207.276481344607));
#26536=CARTESIAN_POINT('',(58.4644314704952,73.2162045685788,207.276481344607));
#26537=CARTESIAN_POINT('',(91.5206923608871,87.0638940383495,207.526481344607));
#26538=CARTESIAN_POINT('Origin',(60.3395802182522,74.2566633166929,202.246481275782));
#26539=CARTESIAN_POINT('',(60.6010403165656,74.0937884510217,197.526481344607));
#26540=CARTESIAN_POINT('',(60.6010403165656,74.0937884510217,197.526481344607));
#26541=CARTESIAN_POINT('',(60.6016091647915,74.0940229189345,197.526481344583));
#26542=CARTESIAN_POINT('',(60.6016091462116,74.09402290755,197.526481344536));
#26543=CARTESIAN_POINT('',(60.7498001670302,74.4136282692967,197.285998169033));
#26544=CARTESIAN_POINT('Ctrl Pts',(60.601609163429,74.0940229222286,197.526481344607));
#26545=CARTESIAN_POINT('Ctrl Pts',(60.6093867240074,74.0972399164823,197.526481344681));
#26546=CARTESIAN_POINT('Ctrl Pts',(60.6170211752848,74.1008569650917,197.526056720543));
#26547=CARTESIAN_POINT('Ctrl Pts',(60.6476006570278,74.1172759128502,197.522566777863));
#26548=CARTESIAN_POINT('Ctrl Pts',(60.6679478441437,74.1328180135862,197.515965357168));
#26549=CARTESIAN_POINT('Ctrl Pts',(60.7071790802335,74.1723286486342,197.494349617611));
#26550=CARTESIAN_POINT('Ctrl Pts',(60.7250505559069,74.1981631566551,197.477205674158));
#26551=CARTESIAN_POINT('Ctrl Pts',(60.7550237921088,74.2639499490842,197.427502643351));
#26552=CARTESIAN_POINT('Ctrl Pts',(60.7631014541665,74.304456312216,197.392855833564));
#26553=CARTESIAN_POINT('Ctrl Pts',(60.7604399586737,74.379903994817,197.321521323378));
#26554=CARTESIAN_POINT('Ctrl Pts',(60.7524970087799,74.4046892292434,197.295405117688));
#26555=CARTESIAN_POINT('Ctrl Pts',(60.7508644926709,74.4101900577452,197.289818721891));
#26556=CARTESIAN_POINT('Ctrl Pts',(60.750542989354,74.411213629704,197.288821964585));
#26557=CARTESIAN_POINT('Ctrl Pts',(60.7500979523006,74.4126077588179,197.287636169735));
#26558=CARTESIAN_POINT('Ctrl Pts',(60.7501077413797,74.412664072175,197.287013854275));
#26559=CARTESIAN_POINT('Ctrl Pts',(60.7498002675722,74.4136280096502,197.285998005213));
#26560=CARTESIAN_POINT('',(60.5926319977064,74.3491829380803,201.741111932353));
#26561=CARTESIAN_POINT('Origin',(94.4639588834092,75.4018623050297,202.246481277241));
#26562=CARTESIAN_POINT('',(94.2048232846065,75.4756444899691,201.741111932351));
#26563=CARTESIAN_POINT('',(94.7093940543517,75.599454730569,207.276481344607));
#26564=CARTESIAN_POINT('Origin',(94.6503106847418,75.3565367291045,207.276481344607));
#26565=CARTESIAN_POINT('',(94.3481720014213,75.6873124271411,197.526481344607));
#26566=CARTESIAN_POINT('',(94.3481720014213,75.6873124271411,197.526481344607));
#26567=CARTESIAN_POINT('',(94.3474637638963,75.6874835959923,197.526481344489));
#26568=CARTESIAN_POINT('Origin',(95.7290969072821,75.0941505546249,183.174071706053));
#26569=CARTESIAN_POINT('',(95.969528519046,75.0256477074975,183.174071706053));
#26570=CARTESIAN_POINT('',(95.788180276892,75.3370685560895,197.526481344607));
#26571=CARTESIAN_POINT('Origin',(95.7290969072821,75.0941505546249,197.526481344607));
#26572=CARTESIAN_POINT('',(95.788180276892,75.3370685560895,197.526481344607));
#26573=CARTESIAN_POINT('Origin',(59.1351724264803,73.7619691814722,183.174071706053));
#26574=CARTESIAN_POINT('',(59.2301565951581,73.5307160567353,197.526481344607));
#26575=CARTESIAN_POINT('',(59.2224992886726,73.5277171395608,197.526481344607));
#26576=CARTESIAN_POINT('Origin',(59.1351724264803,73.7619691814722,197.526481344607));
#26577=CARTESIAN_POINT('',(59.2301565951581,73.5307160567353,197.526481344607));
#26578=CARTESIAN_POINT('',(58.9003582657663,73.6761652775505,197.276481344607));
#26579=CARTESIAN_POINT('',(58.9003582657663,73.6761652775505,183.174071706053));
#26580=CARTESIAN_POINT('Ctrl Pts',(58.9003582657663,73.6761652775505,197.276481344607));
#26581=CARTESIAN_POINT('Ctrl Pts',(58.9006157158184,73.6754607301448,197.277226632397));
#26582=CARTESIAN_POINT('Ctrl Pts',(58.9008763380428,73.6747573380522,197.277971923768));
#26583=CARTESIAN_POINT('Ctrl Pts',(58.9102777590331,73.649730212411,197.304533630725));
#26584=CARTESIAN_POINT('Ctrl Pts',(58.9232676286132,73.6266707314127,197.330483552622));
#26585=CARTESIAN_POINT('Ctrl Pts',(58.9557528174119,73.5860334006603,197.37953436841));
#26586=CARTESIAN_POINT('Ctrl Pts',(58.9751154174747,73.5680078039303,197.403006214922));
#26587=CARTESIAN_POINT('Ctrl Pts',(59.0214638375681,73.5375365062228,197.447428878785));
#26588=CARTESIAN_POINT('Ctrl Pts',(59.0490539838186,73.525140416666,197.468545557742));
#26589=CARTESIAN_POINT('Ctrl Pts',(59.1030897139364,73.5129048458243,197.49872862438));
#26590=CARTESIAN_POINT('Ctrl Pts',(59.1279879313116,73.5107270844252,197.509425478113));
#26591=CARTESIAN_POINT('Ctrl Pts',(59.1764065218,73.5143605752103,197.522897090168));
#26592=CARTESIAN_POINT('Ctrl Pts',(59.1990241075803,73.5191283791597,197.526329043289));
#26593=CARTESIAN_POINT('Ctrl Pts',(59.2215164523983,73.5273525061497,197.526479697129));
#26594=CARTESIAN_POINT('Ctrl Pts',(59.2220082824058,73.5275340972434,197.526481344607));
#26595=CARTESIAN_POINT('Ctrl Pts',(59.2224992886726,73.5277171395608,197.526481344607));
#26596=CARTESIAN_POINT('Origin',(77.215862801455,80.368869783441,197.276481344607));
#26597=CARTESIAN_POINT('',(60.981127142278,73.168836093202,197.526481344546));
#26598=CARTESIAN_POINT('',(61.3110675966908,73.045372688363,197.285998194906));
#26599=CARTESIAN_POINT('Ctrl Pts',(60.9811271425581,73.1688360925134,197.526481344607));
#26600=CARTESIAN_POINT('Ctrl Pts',(60.9971187919203,73.1753416507812,197.526481344728));
#26601=CARTESIAN_POINT('Ctrl Pts',(61.0136652535945,73.180145472812,197.524694774696));
#26602=CARTESIAN_POINT('Ctrl Pts',(61.0582096361667,73.1883912015722,197.515522145646));
#26603=CARTESIAN_POINT('Ctrl Pts',(61.0854542226308,73.1887128146243,197.5055143784));
#26604=CARTESIAN_POINT('Ctrl Pts',(61.1450631440005,73.1810065035281,197.475743629358));
#26605=CARTESIAN_POINT('Ctrl Pts',(61.1779277820307,73.1700125943206,197.453013745431));
#26606=CARTESIAN_POINT('Ctrl Pts',(61.2464250100863,73.1311281924925,197.390673688517));
#26607=CARTESIAN_POINT('Ctrl Pts',(61.2787026839839,73.0999163692651,197.34920192024));
#26608=CARTESIAN_POINT('Ctrl Pts',(61.3060362721128,73.0550865202932,197.296991136723));
#26609=CARTESIAN_POINT('Ctrl Pts',(61.3090465299422,73.0492895571933,197.290418308859));
#26610=CARTESIAN_POINT('Ctrl Pts',(61.310430982896,73.0466070939639,197.287528672697));
#26611=CARTESIAN_POINT('Ctrl Pts',(61.3105752351829,73.0463425312112,197.287089992911));
#26612=CARTESIAN_POINT('Ctrl Pts',(61.3110675074857,73.0453728872428,197.28599813838));
#26613=CARTESIAN_POINT('Origin',(77.215862801455,80.368869783441,197.285998250943));
#26614=CARTESIAN_POINT('Origin',(77.215862801455,80.368869783441,197.526481344607));
#26615=CARTESIAN_POINT('Origin',(94.6503106847418,75.3565367291045,207.276481344607));
#26616=CARTESIAN_POINT('',(94.6503106847418,75.3565367291045,207.526481344607));
#26617=CARTESIAN_POINT('Origin',(94.6503106847418,75.3565367291045,207.276481344607));
#26618=CARTESIAN_POINT('Origin',(94.6503106847418,75.3565367291045,207.276481344607));
#26619=CARTESIAN_POINT('Origin',(77.215862801455,80.368869783441,197.276481344607));
#26620=CARTESIAN_POINT('',(59.602148855249,72.6023016210397,197.526481344607));
#26621=CARTESIAN_POINT('Origin',(77.215862801455,80.368869783441,197.526481344607));
#26622=CARTESIAN_POINT('',(59.4770762970785,72.2703851503661,197.276481344607));
#26623=CARTESIAN_POINT('Origin',(77.215862801455,80.368869783441,197.276481344607));
#26624=CARTESIAN_POINT('Ctrl Pts',(59.4770762970785,72.2703851503661,197.276481344607));
#26625=CARTESIAN_POINT('Ctrl Pts',(59.4767647705069,72.2710675130049,197.277226632396));
#26626=CARTESIAN_POINT('Ctrl Pts',(59.4764563135271,72.2717512810019,197.277971923768));
#26627=CARTESIAN_POINT('Ctrl Pts',(59.4655725732334,72.2961702885867,197.304533630729));
#26628=CARTESIAN_POINT('Ctrl Pts',(59.4586252638423,72.3217087158688,197.330483552621));
#26629=CARTESIAN_POINT('Ctrl Pts',(59.453211504542,72.3734520376809,197.379534368409));
#26630=CARTESIAN_POINT('Ctrl Pts',(59.4543361227423,72.3998824681079,197.403006214921));
#26631=CARTESIAN_POINT('Ctrl Pts',(59.4659309527633,72.4541248495629,197.447428878784));
#26632=CARTESIAN_POINT('Ctrl Pts',(59.4768662169522,72.4823258992516,197.468545557741));
#26633=CARTESIAN_POINT('Ctrl Pts',(59.5067404126769,72.5289853222335,197.498728624379));
#26634=CARTESIAN_POINT('Ctrl Pts',(59.5229356318641,72.5480215705154,197.509425478113));
#26635=CARTESIAN_POINT('Ctrl Pts',(59.5599558615497,72.5794391572182,197.522897090167));
#26636=CARTESIAN_POINT('Ctrl Pts',(59.5794053816239,72.5919292857166,197.526329043289));
#26637=CARTESIAN_POINT('Ctrl Pts',(59.6011931085822,72.6018709553029,197.526479697129));
#26638=CARTESIAN_POINT('Ctrl Pts',(59.6016707655249,72.6020870939782,197.526481344607));
#26639=CARTESIAN_POINT('Ctrl Pts',(59.602148855249,72.6023016210397,197.526481344607));
#26640=CARTESIAN_POINT('Origin',(60.9088619358641,72.8688894817693,202.246481278685));
#26641=CARTESIAN_POINT('',(60.6364778870401,73.0272774920494,207.276481344607));
#26642=CARTESIAN_POINT('Origin',(60.7314620557179,72.7960243673124,207.276481344607));
#26643=CARTESIAN_POINT('',(61.3110676856272,73.0453724901115,197.285998250943));
#26644=CARTESIAN_POINT('',(60.9803477063441,73.1685174815939,197.526481344607));
#26645=CARTESIAN_POINT('',(60.9803477063441,73.1685174815939,197.526481344607));
#26646=CARTESIAN_POINT('',(60.6364778870401,73.0272774920494,207.276481344607));
#26647=CARTESIAN_POINT('Origin',(77.215862801455,80.368869783441,207.276481344607));
#26648=CARTESIAN_POINT('Origin',(77.215862801455,80.368869783441,207.526481344607));
#26649=CARTESIAN_POINT('Origin',(96.135608423356,74.9952773957396,207.276481344607));
#26650=CARTESIAN_POINT('',(95.9862168068599,75.0316129494691,207.526481344607));
#26651=CARTESIAN_POINT('',(96.194691792966,75.2381953972042,207.276481344607));
#26652=CARTESIAN_POINT('Origin',(77.215862801455,80.368869783441,207.276481344607));
#26653=CARTESIAN_POINT('',(79.4109822996944,61.2444364483471,207.526481344607));
#26654=CARTESIAN_POINT('',(79.4394903451261,60.996067184255,207.276481344607));
#26655=CARTESIAN_POINT('Origin',(79.4109822996944,61.2444364483471,207.276481344607));
#26656=CARTESIAN_POINT('Origin',(77.215862801455,80.368869783441,207.276481344607));
#26657=CARTESIAN_POINT('Origin',(77.215862801455,80.368869783441,207.526481344607));
#26658=CARTESIAN_POINT('Origin',(59.7044966368782,72.3742118764312,183.174071706053));
#26659=CARTESIAN_POINT('',(59.6095124682004,72.6054650011681,197.526481344607));
#26660=CARTESIAN_POINT('',(59.6095124682004,72.6054650011681,197.526481344607));
#26661=CARTESIAN_POINT('Origin',(59.7044966368782,72.3742118764312,197.526481344607));
#26662=CARTESIAN_POINT('',(59.4770762970785,72.2703851503661,183.174071706053));
#26663=CARTESIAN_POINT('Origin',(60.7314620557179,72.7960243673124,207.276481344607));
#26664=CARTESIAN_POINT('',(60.7314620557179,72.7960243673124,207.526481344607));
#26665=CARTESIAN_POINT('Origin',(60.7314620557179,72.7960243673124,207.276481344607));
#26666=CARTESIAN_POINT('Origin',(60.7314620557179,72.7960243673124,207.276481344607));
#26667=CARTESIAN_POINT('Origin',(79.4109822996944,61.2444364483471,207.276481344607));
#26668=CARTESIAN_POINT('',(79.1616957861817,61.2255622813273,207.276481344607));
#26669=CARTESIAN_POINT('Origin',(79.4109822996944,61.2444364483471,207.276481344607));
#26670=CARTESIAN_POINT('Origin',(79.4109822996944,61.2444364483471,207.276481344607));
#26671=CARTESIAN_POINT('Origin',(59.0227228960185,72.0941823110984,207.276481344607));
#26672=CARTESIAN_POINT('',(92.090597372954,85.676375289928,207.526481344607));
#26673=CARTESIAN_POINT('',(58.9277387273407,72.3254354358353,207.276481344607));
#26674=CARTESIAN_POINT('Origin',(77.215862801455,80.368869783441,207.276481344607));
#26675=CARTESIAN_POINT('',(77.8314138265035,62.2386587372839,207.526481344607));
#26676=CARTESIAN_POINT('Origin',(77.215862801455,80.368869783441,207.526481344607));
#26677=CARTESIAN_POINT('Origin',(77.8314138265035,62.2386587372839,207.276481344607));
#26678=CARTESIAN_POINT('Origin',(79.3126846293658,62.5427283061288,202.246481278135));
#26679=CARTESIAN_POINT('',(79.269084407634,62.9797812149621,197.285998194441));
#26680=CARTESIAN_POINT('',(79.269084625537,62.9797812385235,197.285998250943));
#26681=CARTESIAN_POINT('',(79.0497526609435,62.7041032964174,197.526481344555));
#26682=CARTESIAN_POINT('Ctrl Pts',(79.2690841890442,62.9797811913385,197.285998137443));
#26683=CARTESIAN_POINT('Ctrl Pts',(79.2680101135346,62.9796124948256,197.28708977948));
#26684=CARTESIAN_POINT('Ctrl Pts',(79.2677145897312,62.9795570615422,197.287528959389));
#26685=CARTESIAN_POINT('Ctrl Pts',(79.2647461981928,62.979070560001,197.290407185081));
#26686=CARTESIAN_POINT('Ctrl Pts',(79.2583629307362,62.9780074907501,197.296918746928));
#26687=CARTESIAN_POINT('Ctrl Pts',(79.2073485996536,62.965904807744,197.349058583512));
#26688=CARTESIAN_POINT('Ctrl Pts',(79.167673145419,62.9448626151971,197.390549949234));
#26689=CARTESIAN_POINT('Ctrl Pts',(79.1094927588433,62.8917379729484,197.452930411033));
#26690=CARTESIAN_POINT('Ctrl Pts',(79.0888676765804,62.8638759507458,197.475678618859));
#26691=CARTESIAN_POINT('Ctrl Pts',(79.0631009548931,62.8095576185035,197.505476436035));
#26692=CARTESIAN_POINT('Ctrl Pts',(79.05498120433,62.7835430926837,197.515495462576));
#26693=CARTESIAN_POINT('Ctrl Pts',(79.0490474931402,62.7385988418192,197.524688969095));
#26694=CARTESIAN_POINT('Ctrl Pts',(79.0485021933496,62.7213503394443,197.526481344716));
#26695=CARTESIAN_POINT('Ctrl Pts',(79.0497526616462,62.7041032964684,197.526481344607));
#26696=CARTESIAN_POINT('',(79.0498116915969,62.7033067469324,197.526481344607));
#26697=CARTESIAN_POINT('',(79.0498116915969,62.7033067469324,197.526481344607));
#26698=CARTESIAN_POINT('',(79.0778774854255,62.3326189234576,207.276481344607));
#26699=CARTESIAN_POINT('Origin',(79.4663159635354,60.513599631853,207.276481344607));
#26700=CARTESIAN_POINT('',(79.2170294500227,60.4947254648331,207.276481344607));
#26701=CARTESIAN_POINT('',(78.4136904864483,74.416482600992,207.526481344607));
#26702=CARTESIAN_POINT('Origin',(79.4109822996944,61.2444364483471,183.174071706053));
#26703=CARTESIAN_POINT('',(79.1624331548021,61.2175417913808,197.526481344607));
#26704=CARTESIAN_POINT('',(79.4394903451261,60.996067184255,197.276481344607));
#26705=CARTESIAN_POINT('Ctrl Pts',(79.1624331548021,61.2175417913808,197.526481344607));
#26706=CARTESIAN_POINT('Ctrl Pts',(79.162489527609,61.2170208175323,197.526481344607));
#26707=CARTESIAN_POINT('Ctrl Pts',(79.1625475669022,61.2164997575336,197.526479697129));
#26708=CARTESIAN_POINT('Ctrl Pts',(79.165273682838,61.1927066885413,197.526329043289));
#26709=CARTESIAN_POINT('Ctrl Pts',(79.1711458432171,61.1703503723531,197.522897090167));
#26710=CARTESIAN_POINT('Ctrl Pts',(79.1895930449751,61.125436422321,197.509425478113));
#26711=CARTESIAN_POINT('Ctrl Pts',(79.2026963979944,61.1041534241107,197.498728624379));
#26712=CARTESIAN_POINT('Ctrl Pts',(79.2378473596214,61.0613284405156,197.468545557741));
#26713=CARTESIAN_POINT('Ctrl Pts',(79.261292025071,61.0422175308465,197.447428878784));
#26714=CARTESIAN_POINT('Ctrl Pts',(79.3093010383479,61.014436050085,197.403006214921));
#26715=CARTESIAN_POINT('Ctrl Pts',(79.3340918218441,61.0052029860052,197.379534368409));
#26716=CARTESIAN_POINT('Ctrl Pts',(79.3849773214833,60.9943703469743,197.330483552621));
#26717=CARTESIAN_POINT('Ctrl Pts',(79.4114128508792,60.9930900494331,197.304533630738));
#26718=CARTESIAN_POINT('Ctrl Pts',(79.4379995190252,60.9958994640783,197.277971923767));
#26719=CARTESIAN_POINT('Ctrl Pts',(79.4387451263528,60.9959816473802,197.277226632397));
#26720=CARTESIAN_POINT('Ctrl Pts',(79.439490345126,60.996067184255,197.276481344607));
#26721=CARTESIAN_POINT('',(79.4394903451261,60.996067184255,183.174071706053));
#26722=CARTESIAN_POINT('',(79.1616957861817,61.2255622813273,197.526481344607));
#26723=CARTESIAN_POINT('',(79.1616957861817,61.2255622813273,197.526481344607));
#26724=CARTESIAN_POINT('Origin',(79.4109822996944,61.2444364483471,197.526481344607));
#26725=CARTESIAN_POINT('Origin',(77.215862801455,80.368869783441,207.276481344607));
#26726=CARTESIAN_POINT('Origin',(77.215862801455,80.368869783441,207.526481344607));
#26727=CARTESIAN_POINT('',(72.6073599718767,61.4212656692062,207.276481344607));
#26728=CARTESIAN_POINT('Origin',(77.215862801455,80.368869783441,207.276481344607));
#26729=CARTESIAN_POINT('Origin',(77.215862801455,80.368869783441,207.276481344607));
#26730=CARTESIAN_POINT('Origin',(77.8314138265035,62.2386587372839,207.276481344607));
#26731=CARTESIAN_POINT('',(78.0807003400161,62.2575329043037,207.276481344607));
#26732=CARTESIAN_POINT('Origin',(77.8314138265035,62.2386587372839,207.276481344607));
#26733=CARTESIAN_POINT('Origin',(77.8314138265035,62.2386587372839,207.276481344607));
#26734=CARTESIAN_POINT('Origin',(77.215862801455,80.368869783441,197.276481344607));
#26735=CARTESIAN_POINT('',(77.7943741989354,62.8685427940256,197.285998169697));
#26736=CARTESIAN_POINT('',(78.052583306941,62.6288859648788,197.526481344578));
#26737=CARTESIAN_POINT('Ctrl Pts',(77.7943744744014,62.8685428093252,197.285998007207));
#26738=CARTESIAN_POINT('Ctrl Pts',(77.7953871004452,62.868537531901,197.287014717876));
#26739=CARTESIAN_POINT('Ctrl Pts',(77.7954406625158,62.868511022385,197.287634888787));
#26740=CARTESIAN_POINT('Ctrl Pts',(77.796910574736,62.8685035682567,197.288828524609));
#26741=CARTESIAN_POINT('Ctrl Pts',(77.7979976652988,62.8684929763872,197.289840350133));
#26742=CARTESIAN_POINT('Ctrl Pts',(77.8029322243904,62.8683662151868,197.294649285739));
#26743=CARTESIAN_POINT('Ctrl Pts',(77.8299951625382,62.868403557902,197.321793962165));
#26744=CARTESIAN_POINT('Ctrl Pts',(77.9036914339881,62.8468136488644,197.394186937533));
#26745=CARTESIAN_POINT('Ctrl Pts',(77.9394990504386,62.8264863037409,197.428597657109));
#26746=CARTESIAN_POINT('Ctrl Pts',(77.9924180066599,62.7775563807812,197.477895540356));
#26747=CARTESIAN_POINT('Ctrl Pts',(78.0113061411039,62.7525744408473,197.494874374673));
#26748=CARTESIAN_POINT('Ctrl Pts',(78.0365242286412,62.7030752536208,197.516246243239));
#26749=CARTESIAN_POINT('Ctrl Pts',(78.0449179730812,62.6789343473944,197.522744141435));
#26750=CARTESIAN_POINT('Ctrl Pts',(78.0509156442943,62.6450929646504,197.526084814193));
#26751=CARTESIAN_POINT('Ctrl Pts',(78.0519478312877,62.6369945577109,197.526481344688));
#26752=CARTESIAN_POINT('Ctrl Pts',(78.052583303161,62.6288859645826,197.526481344607));
#26753=CARTESIAN_POINT('Origin',(77.215862801455,80.368869783441,197.526481344607));
#26754=CARTESIAN_POINT('Origin',(77.215862801455,80.368869783441,197.285998250943));
#26755=CARTESIAN_POINT('Origin',(77.215862801455,80.368869783441,197.276481344607));
#26756=CARTESIAN_POINT('',(78.1650046288044,61.1422832483439,197.526481344607));
#26757=CARTESIAN_POINT('',(77.9243166636283,60.8817434400015,197.276481344607));
#26758=CARTESIAN_POINT('Ctrl Pts',(78.1650046288044,61.1422832483439,197.526481344607));
#26759=CARTESIAN_POINT('Ctrl Pts',(78.16502706682,61.1417597140309,197.526481344607));
#26760=CARTESIAN_POINT('Ctrl Pts',(78.1650478701437,61.1412358444854,197.526479697129));
#26761=CARTESIAN_POINT('Ctrl Pts',(78.1659227895184,61.1173030979625,197.52632904329));
#26762=CARTESIAN_POINT('Ctrl Pts',(78.1634716970727,61.0943187709797,197.522897090169));
#26763=CARTESIAN_POINT('Ctrl Pts',(78.1519727272435,61.047145305419,197.509425478116));
#26764=CARTESIAN_POINT('Ctrl Pts',(78.142211259418,61.0241370977738,197.498728624383));
#26765=CARTESIAN_POINT('Ctrl Pts',(78.1138841938284,60.9765225340547,197.468545557748));
#26766=CARTESIAN_POINT('Ctrl Pts',(78.0935725712605,60.9541101001165,197.447428878792));
#26767=CARTESIAN_POINT('Ctrl Pts',(78.0502757384727,60.9194393588524,197.403006214929));
#26768=CARTESIAN_POINT('Ctrl Pts',(78.0271510587944,60.9065909500587,197.379534368416));
#26769=CARTESIAN_POINT('Ctrl Pts',(77.9784671177831,60.8882455410985,197.330483552625));
#26770=CARTESIAN_POINT('Ctrl Pts',(77.9525229939557,60.8830130642432,197.304533630717));
#26771=CARTESIAN_POINT('Ctrl Pts',(77.9258157775659,60.8818013184771,197.277971923771));
#26772=CARTESIAN_POINT('Ctrl Pts',(77.9250662801213,60.8817706922854,197.277226632395));
#26773=CARTESIAN_POINT('Ctrl Pts',(77.9243166636283,60.8817434400015,197.276481344607));
#26774=CARTESIAN_POINT('Origin',(77.215862801455,80.368869783441,197.276481344607));
#26775=CARTESIAN_POINT('Origin',(77.215862801455,80.368869783441,197.526481344607));
#26776=CARTESIAN_POINT('Origin',(77.9774013323172,60.3104827122258,207.276481344607));
#26777=CARTESIAN_POINT('',(78.2266878458299,60.3293568792457,207.276481344607));
#26778=CARTESIAN_POINT('',(76.9179714053723,74.3032375988726,207.526481344607));
#26779=CARTESIAN_POINT('Origin',(77.8169349762247,62.4298984090937,202.246481276341));
#26780=CARTESIAN_POINT('',(77.8070980354658,62.6991535160838,201.74111193235));
#26781=CARTESIAN_POINT('',(78.0526338951397,62.6282293266983,197.526481344607));
#26782=CARTESIAN_POINT('',(78.0526338951397,62.6282293266983,197.526481344607));
#26783=CARTESIAN_POINT('',(78.0525833124769,62.6288859405896,197.52648134452));
#26784=CARTESIAN_POINT('Origin',(77.9152339218055,61.1315783931226,183.174071706053));
#26785=CARTESIAN_POINT('',(78.1645204353182,61.1504525601425,197.526481344607));
#26786=CARTESIAN_POINT('Origin',(77.9152339218055,61.1315783931226,197.526481344607));
#26787=CARTESIAN_POINT('',(78.1645204353182,61.1504525601425,197.526481344607));
#26788=CARTESIAN_POINT('',(77.9243166636283,60.8817434400015,183.174071706053));
#26789=CARTESIAN_POINT('Origin',(77.215862801455,80.368869783441,194.876481344607));
#26790=CARTESIAN_POINT('',(69.7713582305978,49.7612015989078,194.876481344607));
#26791=CARTESIAN_POINT('Origin',(77.215862801455,80.368869783441,194.876481344607));
#26792=CARTESIAN_POINT('',(69.8304416002078,50.0041196003723,195.126481344607));
#26793=CARTESIAN_POINT('Origin',(69.8304416002078,50.0041196003723,194.876481344607));
#26794=CARTESIAN_POINT('Origin',(77.215862801455,80.368869783441,195.126481344607));
#26795=CARTESIAN_POINT('Origin',(77.215862801455,80.368869783441,197.526481344607));
#26796=CARTESIAN_POINT('',(96.4310252714059,76.2098674030624,197.526481344607));
#26797=CARTESIAN_POINT('',(96.194691792966,75.2381953972042,197.526481344607));
#26798=CARTESIAN_POINT('Origin',(96.194691792966,75.2381953972042,197.526481344607));
#26799=CARTESIAN_POINT('Origin',(96.4310252714059,76.2098674030624,197.526481344607));
#26800=CARTESIAN_POINT('Origin',(78.4583471591332,61.9901304421851,197.526481344607));
#26801=CARTESIAN_POINT('',(79.2170294500227,60.4947254648331,197.526481344607));
#26802=CARTESIAN_POINT('',(78.2266878458299,60.3293568792457,197.526481344607));
#26803=CARTESIAN_POINT('Origin',(79.2170294500227,60.4947254648331,197.526481344607));
#26804=CARTESIAN_POINT('Origin',(78.2266878458299,60.3293568792457,197.526481344607));
#26805=CARTESIAN_POINT('Origin',(60.1155076543353,73.5090907238581,197.526481344607));
#26806=CARTESIAN_POINT('',(58.9277387273407,72.3254354358353,197.526481344607));
#26807=CARTESIAN_POINT('',(58.4644314704952,73.2162045685788,197.526481344607));
#26808=CARTESIAN_POINT('Origin',(58.9277387273407,72.3254354358353,197.526481344607));
#26809=CARTESIAN_POINT('Origin',(58.4644314704952,73.2162045685788,197.526481344607));
#26810=CARTESIAN_POINT('Origin',(65.4024407590908,94.5137222468193,197.526481344607));
#26811=CARTESIAN_POINT('',(63.9096769005376,95.2775880252097,197.526481344607));
#26812=CARTESIAN_POINT('',(64.6136788727654,95.9934822109618,197.526481344607));
#26813=CARTESIAN_POINT('Origin',(63.9096769005376,95.2775880252097,197.526481344607));
#26814=CARTESIAN_POINT('Origin',(64.6136788727654,95.9934822109618,197.526481344607));
#26815=CARTESIAN_POINT('Origin',(87.0127846188746,95.9763381675038,197.526481344607));
#26816=CARTESIAN_POINT('',(87.277974744106,97.6320884694148,197.526481344607));
#26817=CARTESIAN_POINT('',(88.1763791479352,97.1837662758145,197.526481344607));
#26818=CARTESIAN_POINT('Origin',(87.277974744106,97.6320884694148,197.526481344607));
#26819=CARTESIAN_POINT('Origin',(88.1763791479352,97.1837662758145,197.526481344607));
#26820=CARTESIAN_POINT('Origin',(94.9974604855648,76.0439671336079,193.776481344607));
#26821=CARTESIAN_POINT('',(72.8909601516219,62.5872720993312,193.776481344607));
#26822=CARTESIAN_POINT('Origin',(77.215862801455,80.368869783441,193.776481344607));
#26823=CARTESIAN_POINT('Origin',(77.215862801455,80.368869783441,194.576481344607));
#26824=CARTESIAN_POINT('',(73.0800269287566,63.3646096809225,194.576145266601));
#26825=CARTESIAN_POINT('Origin',(77.215862801455,80.368869783441,194.576145266601));
#26826=CARTESIAN_POINT('Origin',(72.890960162688,62.587272144829,194.576481344607));
#26827=CARTESIAN_POINT('Origin',(77.215862801455,80.368869783441,183.174071706053));
#26828=CARTESIAN_POINT('',(73.0800269287565,63.3646096809226,183.174071706053));
#26829=CARTESIAN_POINT('Origin',(77.215862801455,80.368869783441,197.026481344607));
#26830=CARTESIAN_POINT('',(81.3516986741534,97.3731298859594,197.026481344607));
#26831=CARTESIAN_POINT('Origin',(96.1634669156899,75.7603669538627,207.526481344607));
#26832=CARTESIAN_POINT('Origin',(77.215862801455,80.368869783441,183.174071706053));
#26833=CARTESIAN_POINT('',(72.6073599718767,61.4212656692062,183.174071706053));
#26834=CARTESIAN_POINT('Origin',(107.823530985988,72.9243652125838,195.126481344607));
#26835=CARTESIAN_POINT('Origin',(77.215862801455,80.368869783441,183.174071706053));
#26836=CARTESIAN_POINT('',(69.7713582305978,49.7612015989078,183.174071706053));
#26837=CARTESIAN_POINT('Origin',(96.1634669156899,75.7603669538627,207.526481344607));
#26838=CARTESIAN_POINT('Origin',(96.1634669156899,75.7603669538627,207.526481344607));
#26839=CARTESIAN_POINT('Origin',(96.1634669156899,75.7603669538627,207.526481344607));
#26840=CARTESIAN_POINT('Origin',(96.1634669156899,75.7603669538627,207.526481344607));
#36648=UNCERTAINTY_MEASURE_WITH_UNIT(LENGTH_MEASURE(0.01),#36669,
'DISTANCE_ACCURACY_VALUE',
'Maximum model space distance between geometric entities at asserted c
onnectivities');
#36656=UNCERTAINTY_MEASURE_WITH_UNIT(LENGTH_MEASURE(0.01),#36669,
'DISTANCE_ACCURACY_VALUE',
'Maximum model space distance between geometric entities at asserted c
onnectivities');
#36660=(
GEOMETRIC_REPRESENTATION_CONTEXT(3)
GLOBAL_UNCERTAINTY_ASSIGNED_CONTEXT((#36648))
GLOBAL_UNIT_ASSIGNED_CONTEXT((#36669,#36671,#36672))
REPRESENTATION_CONTEXT('','3D')
);
#36668=(
GEOMETRIC_REPRESENTATION_CONTEXT(3)
GLOBAL_UNCERTAINTY_ASSIGNED_CONTEXT((#36656))
GLOBAL_UNIT_ASSIGNED_CONTEXT((#36669,#36671,#36672))
REPRESENTATION_CONTEXT('','3D')
);
#36669=(
LENGTH_UNIT()
NAMED_UNIT(*)
SI_UNIT(.MILLI.,.METRE.)
);
#36671=(
NAMED_UNIT(*)
PLANE_ANGLE_UNIT()
SI_UNIT($,.RADIAN.)
);
#36672=(
NAMED_UNIT(*)
SI_UNIT($,.STERADIAN.)
SOLID_ANGLE_UNIT()
);
#36676=SHAPE_DEFINITION_REPRESENTATION(#36687,#36708);
#36687=PRODUCT_DEFINITION_SHAPE('',$,#36720);
#36708=SHAPE_REPRESENTATION('',(#18270),#36660);
#36716=PRODUCT_DEFINITION_CONTEXT('part definition',#36751,'design');
#36720=PRODUCT_DEFINITION('Cover Tape Peel Off Spool',
'Cover Tape Peel Off Spool',#36731,#36716);
#36731=PRODUCT_DEFINITION_FORMATION('',$,#36756);
#36751=APPLICATION_CONTEXT(
'Core Data for Automotive Mechanical Design Process');
#36752=PRODUCT_CONTEXT('part definition',#36751,'mechanical');
#36756=PRODUCT('Cover Tape Peel Off Spool','Cover Tape Peel Off Spool',
$,(#36752));
#36767=PRESENTATION_STYLE_ASSIGNMENT((#36774));
#36774=SURFACE_STYLE_USAGE(.BOTH.,#36781);
#36781=SURFACE_SIDE_STYLE('',(#36788));
#36788=SURFACE_STYLE_FILL_AREA(#36795);
#36795=FILL_AREA_STYLE('Opaque(185,192,202)',(#36802));
#36802=FILL_AREA_STYLE_COLOUR('Opaque(185,192,202)',#36809);
#36809=COLOUR_RGB('Opaque(185,192,202)',0.725490196078431,0.752941176470588,
0.792156862745098);
ENDSEC;
END-ISO-10303-21;
